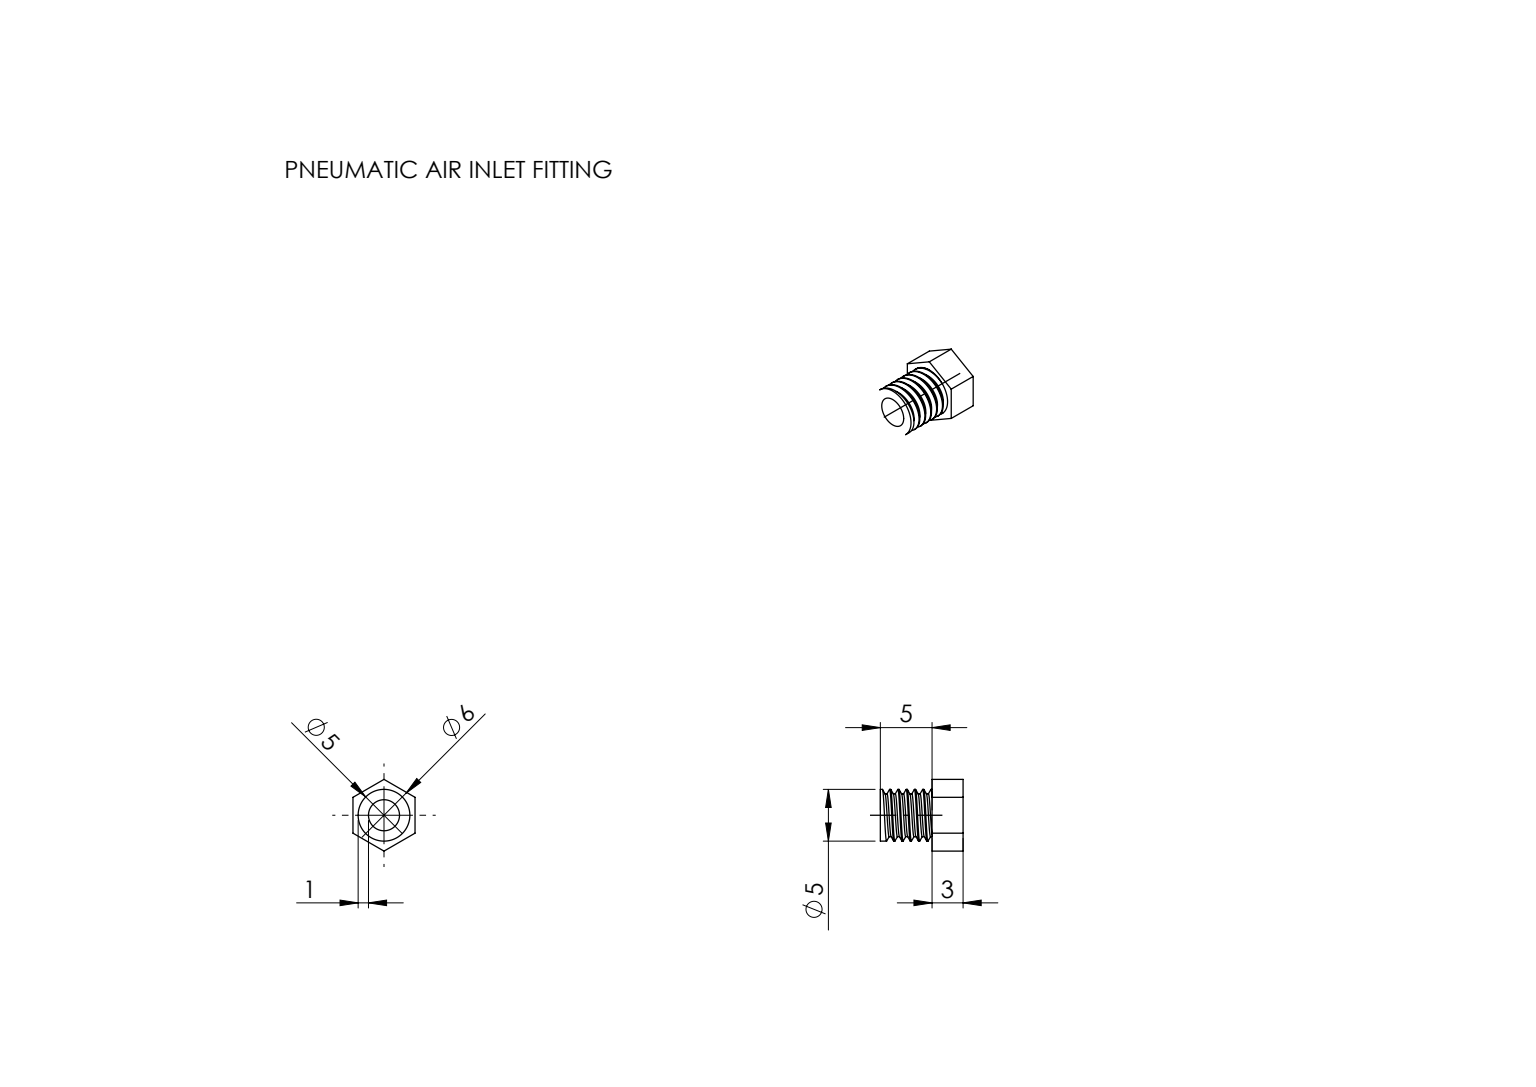
ISO-10303-21;
HEADER;
FILE_DESCRIPTION (('STEP AP214'),
    '1' );
FILE_NAME ('pneumatic air inlet fitting.step',
    '2026-10-04T10:31:01',
    ( '' ),
    ( '' ),
    'SwSTEP 2.0',
    'SolidWorks 2026',
    '' );
FILE_SCHEMA (( 'AUTOMOTIVE_DESIGN' ));
ENDSEC;

DATA;
#1=DIRECTION ( 'NONE',  ( 1.251928832280965695E-16, 1.000000000000000000, 0.000000000000000000 ) ) ;
#9=ORIENTED_EDGE ( 'NONE', *, *, #12350, .T. ) ;
#13=CARTESIAN_POINT ( 'NONE',  ( -1.461580736456472795, 1.461580736456472795, 1.150000001092474688 ) ) ;
#17=CARTESIAN_POINT ( 'NONE',  ( 2.500000000000000000, 3.061616997868383141E-16, 2.100000000000000089 ) ) ;
#21=CARTESIAN_POINT ( 'NONE',  ( 0.8561741729129451750, 2.066987299999999639, 2.000000001092475443 ) ) ;
#26=VERTEX_POINT ( 'NONE', #13779 ) ;
#44=EDGE_LOOP ( 'NONE', ( #13948, #7274 ) ) ;
#48=LINE ( 'NONE', #2436, #232 ) ;
#49=DIRECTION ( 'NONE',  ( -1.000000000000000000, 0.000000000000000000, 0.000000000000000000 ) ) ;
#52=CARTESIAN_POINT ( 'NONE',  ( 1.461580736456473018, -1.461580736456472573, -0.6499999989075253559 ) ) ;
#58=CARTESIAN_POINT ( 'NONE',  ( 0.8561741729129452860, 2.066987299999999639, 2.000000001092474999 ) ) ;
#59=VECTOR ( 'NONE', #8000, 1000.000000000000000 ) ;
#75=CARTESIAN_POINT ( 'NONE',  ( -2.500000000000000000, 0.000000000000000000, -2.199999997815050623 ) ) ;
#81=CARTESIAN_POINT ( 'NONE',  ( 0.000000000000000000, 0.000000000000000000, -5.500000000000000000 ) ) ;
#84=ORIENTED_EDGE ( 'NONE', *, *, #4688, .F. ) ;
#87=ORIENTED_EDGE ( 'NONE', *, *, #14600, .T. ) ;
#88=CARTESIAN_POINT ( 'NONE',  ( -1.035533905932737753, 2.500000000000000444, -1.549999997815050490 ) ) ;
#93=AXIS2_PLACEMENT_3D ( 'NONE', #6041, #2604, #1097 ) ;
#94=CARTESIAN_POINT ( 'NONE',  ( -1.530808498934191571E-16, 2.500000000000000000, 0.6999999999999998446 ) ) ;
#98=CARTESIAN_POINT ( 'NONE',  ( 2.066987299999999639, 0.8561741729129456191, -2.299999998907525711 ) ) ;
#101=DIRECTION ( 'NONE',  ( 0.000000000000000000, 0.000000000000000000, -1.000000000000000000 ) ) ;
#129=CARTESIAN_POINT ( 'NONE',  ( 3.796994071234844259E-16, -2.066987299999999639, 0.8500000010924748661 ) ) ;
#134=CARTESIAN_POINT ( 'NONE',  ( -2.500000000000000000, 0.000000000000000000, -2.199999997815050623 ) ) ;
#136=CARTESIAN_POINT ( 'NONE',  ( 0.8561741729129452860, 2.066987299999999639, -1.199999998907525178 ) ) ;
#139=CARTESIAN_POINT ( 'NONE',  ( 0.8561741729129465073, -2.066987299999999195, 0.7000000010924749549 ) ) ;
#167=CARTESIAN_POINT ( 'NONE',  ( -1.461580736456472351, -1.461580736456473018, -0.2499999989075251672 ) ) ;
#171=CARTESIAN_POINT ( 'NONE',  ( 1.767766952966369320, -1.767766952966368654, 2.000000000000000000 ) ) ;
#175=CARTESIAN_POINT ( 'NONE',  ( 2.066987300000000083, -0.8561741729129449530, -0.7999999989075252671 ) ) ;
#180=ORIENTED_EDGE ( 'NONE', *, *, #12545, .T. ) ;
#187=DIRECTION ( 'NONE',  ( 0.8660254037844385966, 0.4999999999999998890, 0.000000000000000000 ) ) ;
#201=EDGE_CURVE ( 'NONE', #13777, #13408, #2146, .T. ) ;
#202=VERTEX_POINT ( 'NONE', #2611 ) ;
#209=( BOUNDED_CURVE ( )  B_SPLINE_CURVE ( 2, ( #7437, #5274, #15205, #1752, #11093, #14680, #10274, #6626, #3769 ),
 .UNSPECIFIED., .F., .F. ) 
 B_SPLINE_CURVE_WITH_KNOTS ( ( 3, 2, 2, 2, 3 ),
 ( 0.000000000000000000, 0.01785714285714285615, 0.03571428571428571230, 0.05357142857142856845, 0.07142857142857142461 ),
 .UNSPECIFIED. ) 
 CURVE ( )  GEOMETRIC_REPRESENTATION_ITEM ( )  RATIONAL_B_SPLINE_CURVE ( ( 1.000000000000000000, 0.9238795325112867385, 1.000000000000000000, 0.9238795325112867385, 1.000000000000000000, 0.9238795325112867385, 1.000000000000000000, 0.9238795325112867385, 1.000000000000000000 ) ) 
 REPRESENTATION_ITEM ( '' )  );
#213=CARTESIAN_POINT ( 'NONE',  ( 0.8561741729129451750, 2.066987299999999639, -1.199999998907525622 ) ) ;
#220=CARTESIAN_POINT ( 'NONE',  ( -0.8561741729129455081, 2.066987299999999639, -1.899999998907525134 ) ) ;
#222=CARTESIAN_POINT ( 'NONE',  ( -1.265664690411614835E-16, 2.066987299999999639, 0.2500000010924746663 ) ) ;
#232=VECTOR ( 'NONE', #9608, 1000.000000000000000 ) ;
#248=CARTESIAN_POINT ( 'NONE',  ( 3.796994071234844259E-16, -2.066987299999999639, -0.1499999989075253282 ) ) ;
#252=CARTESIAN_POINT ( 'NONE',  ( 0.4831378333609244180, 2.500000000000000000, -2.516327958217759342 ) ) ;
#256=CARTESIAN_POINT ( 'NONE',  ( 3.796994071234844259E-16, -2.066987299999999639, 0.8500000010924748661 ) ) ;
#286=CARTESIAN_POINT ( 'NONE',  ( -0.8561741729129455081, 2.066987299999999639, -1.899999998907525134 ) ) ;
#289=ADVANCED_FACE ( 'NONE', ( #4509 ), #10713, .T. ) ;
#294=LINE ( 'NONE', #13810, #11835 ) ;
#325=CARTESIAN_POINT ( 'NONE',  ( -2.066987299999999639, 0.8561741729129452860, 0.4000000010924749105 ) ) ;
#326=CARTESIAN_POINT ( 'NONE',  ( -1.767766952966369098, 1.767766952966369098, -1.600000000000000311 ) ) ;
#329=CARTESIAN_POINT ( 'NONE',  ( -2.500000000000000444, 1.035533905932737753, 0.05000000000000014155 ) ) ;
#333=CARTESIAN_POINT ( 'NONE',  ( 0.8561741729129451750, 2.066987299999999639, -1.199999998907525622 ) ) ;
#338=VERTEX_POINT ( 'NONE', #15412 ) ;
#355=EDGE_CURVE ( 'NONE', #9607, #3437, #6727, .T. ) ;
#360=CARTESIAN_POINT ( 'NONE',  ( -2.500000000000000000, 0.000000000000000000, 1.700000000000000178 ) ) ;
#366=CARTESIAN_POINT ( 'NONE',  ( -1.265664690411614835E-16, 2.066987299999999639, -1.149999998907525356 ) ) ;
#372=CARTESIAN_POINT ( 'NONE',  ( 2.066987300000000083, -0.8561741729129450640, -1.399999998907525134 ) ) ;
#373=CARTESIAN_POINT ( 'NONE',  ( 2.500000000000000000, 3.061616997868383141E-16, -2.599999997815050534 ) ) ;
#374=CARTESIAN_POINT ( 'NONE',  ( 0.8561741729129452860, 2.066987299999999639, 1.800000001092475044 ) ) ;
#379=CARTESIAN_POINT ( 'NONE',  ( 2.500000000000000000, 3.061616997868383141E-16, -0.2999999999999999334 ) ) ;
#399=CARTESIAN_POINT ( 'NONE',  ( 2.066987299999999639, 0.8561741729129456191, -2.299999998907525711 ) ) ;
#403=CARTESIAN_POINT ( 'NONE',  ( -2.500000000000000000, 0.000000000000000000, 1.800000002184949821 ) ) ;
#406=CARTESIAN_POINT ( 'NONE',  ( 1.035533905932737531, 2.500000000000000444, -0.8499999978150500901 ) ) ;
#407=CARTESIAN_POINT ( 'NONE',  ( 3.796994071234844259E-16, -2.066987299999999639, 0.05000000109247476621 ) ) ;
#408=( BOUNDED_CURVE ( )  B_SPLINE_CURVE ( 2, ( #13845, #5357, #15207, #15052, #7888, #406, #8045, #8938, #10125 ),
 .UNSPECIFIED., .F., .F. ) 
 B_SPLINE_CURVE_WITH_KNOTS ( ( 3, 2, 2, 2, 3 ),
 ( 0.4285714285714285476, 0.4464285714285714524, 0.4642857142857143016, 0.4821428571428571508, 0.5000000000000000000 ),
 .UNSPECIFIED. ) 
 CURVE ( )  GEOMETRIC_REPRESENTATION_ITEM ( )  RATIONAL_B_SPLINE_CURVE ( ( 1.000000000000000000, 0.9238795325112867385, 1.000000000000000000, 0.9238795325112867385, 1.000000000000000000, 0.9238795325112867385, 1.000000000000000000, 0.9238795325112867385, 1.000000000000000000 ) ) 
 REPRESENTATION_ITEM ( '' )  );
#412=EDGE_LOOP ( 'NONE', ( #8229, #15228, #15119, #15116 ) ) ;
#413=VECTOR ( 'NONE', #15523, 1000.000000000000000 ) ;
#439=CARTESIAN_POINT ( 'NONE',  ( 1.035533905932737531, 2.500000000000000444, 1.450000000000000400 ) ) ;
#477=APPLICATION_CONTEXT ( 'automotive_design' ) ;
#480=CARTESIAN_POINT ( 'NONE',  ( 2.066987300000000083, -0.8561741729129449530, -2.399999998907525356 ) ) ;
#483=CARTESIAN_POINT ( 'NONE',  ( 1.767766952966369320, -1.767766952966368654, -0.4000000000000001887 ) ) ;
#487=CARTESIAN_POINT ( 'NONE',  ( -1.265664690411614835E-16, 2.066987299999999639, -1.149999998907525356 ) ) ;
#503=CARTESIAN_POINT ( 'NONE',  ( 1.767766952966369320, -1.767766952966368654, -2.000000000000000444 ) ) ;
#510=CARTESIAN_POINT ( 'NONE',  ( -2.055837405312323174, -1.429616716009805888, -2.499172079278979997 ) ) ;
#519=CARTESIAN_POINT ( 'NONE',  ( 1.461580736456472573, 1.461580736456472795, -1.249999998907525223 ) ) ;
#528=CARTESIAN_POINT ( 'NONE',  ( -0.8561741729129458411, -2.066987299999999195, -1.799999998907525045 ) ) ;
#546=VERTEX_POINT ( 'NONE', #7374 ) ;
#553=EDGE_CURVE ( 'NONE', #3385, #10225, #2858, .T. ) ;
#556=CARTESIAN_POINT ( 'NONE',  ( -3.000000000000000444, -1.732050807568878081, -5.500000000000000000 ) ) ;
#560=CARTESIAN_POINT ( 'NONE',  ( -1.035533905932737753, 2.500000000000000444, -0.05000000000000014155 ) ) ;
#564=DIRECTION ( 'NONE',  ( 0.000000000000000000, 0.000000000000000000, 1.000000000000000000 ) ) ;
#565=CARTESIAN_POINT ( 'NONE',  ( -1.461580736456472795, 1.461580736456472795, -0.2499999989075251672 ) ) ;
#573=ORIENTED_EDGE ( 'NONE', *, *, #355, .F. ) ;
#575=CARTESIAN_POINT ( 'NONE',  ( 1.035533905932739085, -2.500000000000000000, 0.4500000021849495657 ) ) ;
#587=EDGE_LOOP ( 'NONE', ( #4059, #13067, #6384, #6203 ) ) ;
#598=CARTESIAN_POINT ( 'NONE',  ( -2.500000000000000000, -1.035533905932739307, -0.6500000000000000222 ) ) ;
#605=CARTESIAN_POINT ( 'NONE',  ( 2.066987299999999639, 2.531329380823229670E-16, -1.549999998907525489 ) ) ;
#631=DIRECTION ( 'NONE',  ( -0.8660254037844387076, -0.4999999999999998890, 0.000000000000000000 ) ) ;
#632=CARTESIAN_POINT ( 'NONE',  ( 1.035533905932737531, 2.500000000000000444, -1.750000000000000222 ) ) ;
#646=CARTESIAN_POINT ( 'NONE',  ( 4.592425496802573972E-16, -2.500000000000000000, 0.4000000021849496878 ) ) ;
#654=CARTESIAN_POINT ( 'NONE',  ( -1.265664690411614835E-16, 2.066987299999999639, 1.850000001092474644 ) ) ;
#659=CARTESIAN_POINT ( 'NONE',  ( 2.356441885422377425, -0.8834023615831587684, -2.499692266475796121 ) ) ;
#669=CARTESIAN_POINT ( 'NONE',  ( 1.035533905932739085, -2.500000000000000000, -0.4499999999999998446 ) ) ;
#679=CARTESIAN_POINT ( 'NONE',  ( -2.066987299999999195, -0.8561741729129467293, -1.099999998907525312 ) ) ;
#685=ORIENTED_EDGE ( 'NONE', *, *, #2400, .T. ) ;
#707=CARTESIAN_POINT ( 'NONE',  ( -0.8561741729129458411, -2.066987299999999195, -2.599999998907525534 ) ) ;
#713=CARTESIAN_POINT ( 'NONE',  ( 4.592425496802573972E-16, -2.500000000000000000, -0.5000000000000000000 ) ) ;
#715=CARTESIAN_POINT ( 'NONE',  ( 2.500000000000000000, 3.061616997868383141E-16, -1.799999997815050490 ) ) ;
#720=ADVANCED_FACE ( 'NONE', ( #5682 ), #7733, .T. ) ;
#726=PLANE ( 'NONE',  #3772 ) ;
#730=CARTESIAN_POINT ( 'NONE',  ( -2.500000000000000444, 1.035533905932737753, 0.1500000021849496601 ) ) ;
#735=CARTESIAN_POINT ( 'NONE',  ( -2.500000000000000000, 0.000000000000000000, 1.706999999978150662 ) ) ;
#737=SHAPE_DEFINITION_REPRESENTATION ( #15269, #5305 ) ;
#739=CARTESIAN_POINT ( 'NONE',  ( -1.265664690411614835E-16, 2.066987299999999639, 0.2500000010924746663 ) ) ;
#743=CARTESIAN_POINT ( 'NONE',  ( -1.530808498934191571E-16, 2.500000000000000000, 0.8000000021849498211 ) ) ;
#745=CARTESIAN_POINT ( 'NONE',  ( -2.135032056815611146, -1.308652412870009663, -2.499304978889202555 ) ) ;
#753=CARTESIAN_POINT ( 'NONE',  ( 0.3272492347489360798, 2.500000000000000000, -2.500000000000000000 ) ) ;
#755=CARTESIAN_POINT ( 'NONE',  ( 2.500000000000000444, 1.035533905932737975, -1.850000000000000533 ) ) ;
#765=CARTESIAN_POINT ( 'NONE',  ( 1.461580736456473018, -1.461580736456472573, -0.04999999890752549608 ) ) ;
#771=EDGE_CURVE ( 'NONE', #5999, #10225, #9169, .T. ) ;
#776=CARTESIAN_POINT ( 'NONE',  ( 4.592425496802573972E-16, -2.500000000000000000, -0.3999999978150502455 ) ) ;
#782=CARTESIAN_POINT ( 'NONE',  ( -1.035533905932738197, -2.500000000000000000, 1.150000002184949466 ) ) ;
#786=VERTEX_POINT ( 'NONE', #4622 ) ;
#794=CARTESIAN_POINT ( 'NONE',  ( -2.500000000000000000, -1.035533905932739307, -0.5499999978150503788 ) ) ;
#801=ORIENTED_EDGE ( 'NONE', *, *, #1804, .T. ) ;
#805=PLANE ( 'NONE',  #9364 ) ;
#808=CARTESIAN_POINT ( 'NONE',  ( 2.500000000000000000, 3.061616997868383141E-16, 0.6000000021849495324 ) ) ;
#812=CARTESIAN_POINT ( 'NONE',  ( -1.530808498934191571E-16, 2.500000000000000000, -1.693000000021849916 ) ) ;
#815=CARTESIAN_POINT ( 'NONE',  ( -1.265664690411614835E-16, 2.066987299999999639, 1.050000001092474822 ) ) ;
#822=CARTESIAN_POINT ( 'NONE',  ( -2.397391504966196241, 0.7648662538461182825, -2.499399845735361225 ) ) ;
#833=CARTESIAN_POINT ( 'NONE',  ( 2.500000000000000444, 1.035533905932737975, 0.5499999999999999334 ) ) ;
#836=( BOUNDED_CURVE ( )  B_SPLINE_CURVE ( 2, ( #3676, #14327, #3434, #8554, #13378 ),
 .UNSPECIFIED., .F., .F. ) 
 B_SPLINE_CURVE_WITH_KNOTS ( ( 3, 2, 3 ),
 ( 0.8571428571428570953, 0.8750000000000000000, 0.8928571428571429047 ),
 .UNSPECIFIED. ) 
 CURVE ( )  GEOMETRIC_REPRESENTATION_ITEM ( )  RATIONAL_B_SPLINE_CURVE ( ( 1.000000000000000000, 0.9238795325112867385, 1.000000000000000000, 0.9238795325112867385, 1.000000000000000000 ) ) 
 REPRESENTATION_ITEM ( '' )  );
#848=CARTESIAN_POINT ( 'NONE',  ( 0.000000000000000000, 0.000000000000000000, 2.500000000000000000 ) ) ;
#870=CARTESIAN_POINT ( 'NONE',  ( -1.035533905932738197, -2.500000000000000000, 1.150000002184949466 ) ) ;
#873=CARTESIAN_POINT ( 'NONE',  ( -2.500000000000000000, 0.000000000000000000, 0.9000000000000000222 ) ) ;
#879=ORIENTED_EDGE ( 'NONE', *, *, #5328, .F. ) ;
#883=CARTESIAN_POINT ( 'NONE',  ( -2.500000000000000000, -1.035533905932739307, -0.5499999978150504898 ) ) ;
#887=CARTESIAN_POINT ( 'NONE',  ( 1.035533905932739085, -2.500000000000000000, -0.4430000000218494716 ) ) ;
#890=CARTESIAN_POINT ( 'NONE',  ( 1.461580736456473018, -1.461580736456472573, 1.550000001092474822 ) ) ;
#900=LINE ( 'NONE', #8075, #8869 ) ;
#908=CARTESIAN_POINT ( 'NONE',  ( -2.500000000000000000, -1.035533905932739307, 0.9499999999999999556 ) ) ;
#914=( BOUNDED_CURVE ( )  B_SPLINE_CURVE ( 2, ( #2367, #1402, #6046, #2449, #8594, #10887, #8350, #11039, #13269 ),
 .UNSPECIFIED., .F., .F. ) 
 B_SPLINE_CURVE_WITH_KNOTS ( ( 3, 2, 2, 2, 3 ),
 ( 0.1428571428571428492, 0.1607142857142857262, 0.1785714285714285754, 0.1964285714285714246, 0.2142857142857142738 ),
 .UNSPECIFIED. ) 
 CURVE ( )  GEOMETRIC_REPRESENTATION_ITEM ( )  RATIONAL_B_SPLINE_CURVE ( ( 1.000000000000000000, 0.9238795325112867385, 1.000000000000000000, 0.9238795325112867385, 1.000000000000000000, 0.9238795325112867385, 1.000000000000000000, 0.9238795325112867385, 1.000000000000000000 ) ) 
 REPRESENTATION_ITEM ( '' )  );
#922=ORIENTED_EDGE ( 'NONE', *, *, #11635, .F. ) ;
#930=AXIS2_PLACEMENT_3D ( 'NONE', #4602, #8185, #8263 ) ;
#933=CARTESIAN_POINT ( 'NONE',  ( 1.461580736456473018, -1.461580736456472573, 1.750000001092474999 ) ) ;
#941=ORIENTED_EDGE ( 'NONE', *, *, #5328, .T. ) ;
#948=FACE_OUTER_BOUND ( 'NONE', #587, .T. ) ;
#949=CARTESIAN_POINT ( 'NONE',  ( -2.500000000000000444, 1.035533905932737753, -0.6499999978150502455 ) ) ;
#953=CARTESIAN_POINT ( 'NONE',  ( -1.767766952966369098, 1.767766952966369098, 0.7999999999999999334 ) ) ;
#964=CARTESIAN_POINT ( 'NONE',  ( 2.066987300000000083, -0.8561741729129449530, 1.600000001092474644 ) ) ;
#969=CARTESIAN_POINT ( 'NONE',  ( -1.530808498934191571E-16, 2.500000000000000000, -0.8930000000218497602 ) ) ;
#972=CARTESIAN_POINT ( 'NONE',  ( 0.8561741729129463963, -2.066987299999999195, 1.500000001092474555 ) ) ;
#987=CYLINDRICAL_SURFACE ( 'NONE', #1712, 2.500000000000000000 ) ;
#1003=CARTESIAN_POINT ( 'NONE',  ( -1.767766952966369098, 1.767766952966369098, -1.499999997815050001 ) ) ;
#1009=CARTESIAN_POINT ( 'NONE',  ( -2.066987299999999639, 0.8561741729129452860, 1.400000001092474911 ) ) ;
#1017=CARTESIAN_POINT ( 'NONE',  ( -1.461580736456472795, 1.461580736456472795, -1.049999998907525045 ) ) ;
#1018=CARTESIAN_POINT ( 'NONE',  ( -2.500000000000000000, 0.000000000000000000, -1.399999997815050357 ) ) ;
#1029=CARTESIAN_POINT ( 'NONE',  ( 1.035533905932737531, 2.500000000000000444, -1.649999997815050357 ) ) ;
#1045=CARTESIAN_POINT ( 'NONE',  ( -2.500000000000000444, 1.035533905932737753, -1.449999997815050623 ) ) ;
#1049=CARTESIAN_POINT ( 'NONE',  ( 1.035533905932737531, 2.500000000000000444, -0.9430000000218496936 ) ) ;
#1052=CARTESIAN_POINT ( 'NONE',  ( -1.265664690411614835E-16, 2.066987299999999639, -2.149999998907525800 ) ) ;
#1057=VECTOR ( 'NONE', #10344, 1000.000000000000000 ) ;
#1084=CARTESIAN_POINT ( 'NONE',  ( 2.500000000000000000, 3.061616997868383141E-16, -1.100000000000000311 ) ) ;
#1089=CARTESIAN_POINT ( 'NONE',  ( 1.461580736456472573, 1.461580736456472795, 1.150000001092474911 ) ) ;
#1096=CARTESIAN_POINT ( 'NONE',  ( -2.066987299999999195, -0.8561741729129467293, 1.500000001092474777 ) ) ;
#1097=DIRECTION ( 'NONE',  ( -1.000000000000000000, 0.000000000000000000, 0.000000000000000000 ) ) ;
#1110=CARTESIAN_POINT ( 'NONE',  ( -2.500000000000000444, 1.035533905932737753, 0.9500000021849498433 ) ) ;
#1122=CARTESIAN_POINT ( 'NONE',  ( -1.265664690411614835E-16, 2.066987299999999639, 1.050000001092474822 ) ) ;
#1126=CARTESIAN_POINT ( 'NONE',  ( -1.767766952966369098, 1.767766952966369098, 0.006999999978150502240 ) ) ;
#1129=CARTESIAN_POINT ( 'NONE',  ( -1.461580736456472351, -1.461580736456473018, -2.649999998907525356 ) ) ;
#1134=ORIENTED_EDGE ( 'NONE', *, *, #3829, .F. ) ;
#1143=EDGE_CURVE ( 'NONE', #8784, #13466, #6997, .T. ) ;
#1163=CARTESIAN_POINT ( 'NONE',  ( 2.066987300000000083, -0.8561741729129449530, 0.2000000010924747329 ) ) ;
#1171=CARTESIAN_POINT ( 'NONE',  ( -2.066987299999999639, 0.000000000000000000, -0.1499999989075253282 ) ) ;
#1191=ORIENTED_EDGE ( 'NONE', *, *, #15384, .T. ) ;
#1197=CARTESIAN_POINT ( 'NONE',  ( -1.767766952966369098, 1.767766952966369098, -3.099999997815050090 ) ) ;
#1202=CARTESIAN_POINT ( 'NONE',  ( 1.035533905932739085, -2.500000000000000000, 1.949999999999999956 ) ) ;
#1206=CARTESIAN_POINT ( 'NONE',  ( 1.461580736456472573, 1.461580736456472795, -1.449999998907525178 ) ) ;
#1214=VERTEX_POINT ( 'NONE', #12948 ) ;
#1219=DIRECTION ( 'NONE',  ( 0.5000000000000001110, 0.8660254037844385966, 0.000000000000000000 ) ) ;
#1223=CARTESIAN_POINT ( 'NONE',  ( 0.000000000000000000, 0.000000000000000000, 2.500000000000000000 ) ) ;
#1242=EDGE_CURVE ( 'NONE', #5900, #7812, #3452, .T. ) ;
#1244=CARTESIAN_POINT ( 'NONE',  ( -0.8561741729129458411, -2.066987299999999195, -0.7999999989075252671 ) ) ;
#1250=CARTESIAN_POINT ( 'NONE',  ( 1.461580736456472573, 1.461580736456472795, 0.3500000010924749216 ) ) ;
#1259=VECTOR ( 'NONE', #15235, 1000.000000000000227 ) ;
#1264=CARTESIAN_POINT ( 'NONE',  ( -2.500000000000000444, 1.035533905932737753, -3.049999997815050268 ) ) ;
#1270=ORIENTED_EDGE ( 'NONE', *, *, #12295, .F. ) ;
#1273=ORIENTED_EDGE ( 'NONE', *, *, #3458, .F. ) ;
#1274=EDGE_CURVE ( 'NONE', #2475, #11794, #294, .T. ) ;
#1278=CARTESIAN_POINT ( 'NONE',  ( 2.500000000000000000, 3.061616997868383141E-16, -2.599999997815050534 ) ) ;
#1282=CARTESIAN_POINT ( 'NONE',  ( 2.500000000000000444, 1.035533905932737975, 2.149999999999999911 ) ) ;
#1286=CARTESIAN_POINT ( 'NONE',  ( 1.461580736456473018, -1.461580736456472573, -2.449999998907525622 ) ) ;
#1290=VERTEX_POINT ( 'NONE', #6516 ) ;
#1318=CARTESIAN_POINT ( 'NONE',  ( 2.066987299999999639, 2.531329380823229670E-16, 1.850000001092474866 ) ) ;
#1320=ADVANCED_FACE ( 'NONE', ( #2764, #8667 ), #14937, .F. ) ;
#1321=LINE ( 'NONE', #6197, #2164 ) ;
#1326=CARTESIAN_POINT ( 'NONE',  ( -0.8561741729129455081, 2.066987299999999639, -2.699999998907525622 ) ) ;
#1343=CARTESIAN_POINT ( 'NONE',  ( -2.500000000000000000, 0.000000000000000000, -2.999999997815050889 ) ) ;
#1344=DIRECTION ( 'NONE',  ( 0.000000000000000000, 0.000000000000000000, 1.000000000000000000 ) ) ;
#1351=EDGE_LOOP ( 'NONE', ( #3419, #1134, #3681, #13778, #10714 ) ) ;
#1356=CARTESIAN_POINT ( 'NONE',  ( -1.461580736456472795, 1.461580736456472795, 0.3500000010924746996 ) ) ;
#1361=CARTESIAN_POINT ( 'NONE',  ( -1.035533905932737753, 2.500000000000000444, 1.550000000000000044 ) ) ;
#1365=CARTESIAN_POINT ( 'NONE',  ( -0.8561741729129458411, -2.066987299999999195, -0.9999999989075254447 ) ) ;
#1387=ORIENTED_EDGE ( 'NONE', *, *, #10097, .T. ) ;
#1390=CARTESIAN_POINT ( 'NONE',  ( -1.530808498934191571E-16, 2.500000000000000000, -0.9000000000000002442 ) ) ;
#1394=CARTESIAN_POINT ( 'NONE',  ( -1.461580736456472351, -1.461580736456473018, -2.449999998907525178 ) ) ;
#1402=CARTESIAN_POINT ( 'NONE',  ( -2.500000000000000444, 1.035533905932737753, 1.649999999999999911 ) ) ;
#1417=LINE ( 'NONE', #14557, #14169 ) ;
#1425=( BOUNDED_CURVE ( )  B_SPLINE_CURVE ( 2, ( #5701, #11576, #12925, #9201, #13963, #3070, #14041, #7921, #15403 ),
 .UNSPECIFIED., .F., .F. ) 
 B_SPLINE_CURVE_WITH_KNOTS ( ( 3, 2, 2, 2, 3 ),
 ( 0.000000000000000000, 0.01785714285714285615, 0.03571428571428571230, 0.05357142857142856845, 0.07142857142857142461 ),
 .UNSPECIFIED. ) 
 CURVE ( )  GEOMETRIC_REPRESENTATION_ITEM ( )  RATIONAL_B_SPLINE_CURVE ( ( 1.000000000000000000, 0.9238795325112867385, 1.000000000000000000, 0.9238795325112867385, 1.000000000000000000, 0.9238795325112867385, 1.000000000000000000, 0.9238795325112867385, 1.000000000000000000 ) ) 
 REPRESENTATION_ITEM ( '' )  );
#1431=CARTESIAN_POINT ( 'NONE',  ( 0.8561741729129451750, 2.066987299999999639, -1.399999998907525800 ) ) ;
#1436=CARTESIAN_POINT ( 'NONE',  ( -2.500000000000000444, 1.035533905932737753, 2.449999999999999734 ) ) ;
#1439=CARTESIAN_POINT ( 'NONE',  ( -2.066987299999999639, 0.8561741729129452860, 0.6000000010924748661 ) ) ;
#1475=CARTESIAN_POINT ( 'NONE',  ( -2.066987299999999639, 0.8561741729129452860, -1.799999998907525267 ) ) ;
#1479=CARTESIAN_POINT ( 'NONE',  ( -2.283493650000000041, 0.000000000000000000, 2.375000000546237278 ) ) ;
#1481=CARTESIAN_POINT ( 'NONE',  ( 0.8561741729129452860, 2.066987299999999639, -1.999999998907525445 ) ) ;
#1482=CARTESIAN_POINT ( 'NONE',  ( -1.035533905932737753, 2.500000000000000444, -3.149999997815050801 ) ) ;
#1483=CARTESIAN_POINT ( 'NONE',  ( -2.066987299999999639, 0.000000000000000000, 2.050000001092474822 ) ) ;
#1513=CARTESIAN_POINT ( 'NONE',  ( -0.8561741729129458411, -2.066987299999999195, -0.9999999989075254447 ) ) ;
#1517=CARTESIAN_POINT ( 'NONE',  ( -2.500000000000000000, 0.000000000000000000, 0.09999999999999982514 ) ) ;
#1520=MECHANICAL_DESIGN_GEOMETRIC_PRESENTATION_REPRESENTATION('',(#15246),#9915);
#1522=CARTESIAN_POINT ( 'NONE',  ( 2.066987299999999639, 2.531329380823229670E-16, -0.5499999989075250451 ) ) ;
#1556=CARTESIAN_POINT ( 'NONE',  ( 1.035533905932739085, -2.500000000000000000, 1.150000000000000133 ) ) ;
#1563=CARTESIAN_POINT ( 'NONE',  ( 0.000000000000000000, 0.000000000000000000, -2.500000000000000000 ) ) ;
#1565=CARTESIAN_POINT ( 'NONE',  ( -1.767766952966368432, -1.767766952966369320, -2.899999997815050357 ) ) ;
#1566=CARTESIAN_POINT ( 'NONE',  ( 2.066987300000000083, -0.8561741729129450640, 1.092474635061568626E-09 ) ) ;
#1570=VERTEX_POINT ( 'NONE', #10257 ) ;
#1575=CARTESIAN_POINT ( 'NONE',  ( -2.500000000000000000, 0.000000000000000000, 0.09999999999999982514 ) ) ;
#1591=CARTESIAN_POINT ( 'NONE',  ( 0.8561741729129451750, 2.066987299999999639, -2.199999998907525622 ) ) ;
#1595=CARTESIAN_POINT ( 'NONE',  ( 0.9662756667218489470, 2.500000000000000000, -2.546655916391819652 ) ) ;
#1598=CARTESIAN_POINT ( 'NONE',  ( -1.461580736456472795, 1.461580736456472795, 0.5500000010924748217 ) ) ;
#1603=ORIENTED_EDGE ( 'NONE', *, *, #7772, .F. ) ;
#1616=CARTESIAN_POINT ( 'NONE',  ( 2.500000000000000444, 1.035533905932737975, 1.356999999978150573 ) ) ;
#1624=ORIENTED_EDGE ( 'NONE', *, *, #4651, .T. ) ;
#1633=CARTESIAN_POINT ( 'NONE',  ( 1.767766952966369320, -1.767766952966368654, 2.000000000000000000 ) ) ;
#1636=CARTESIAN_POINT ( 'NONE',  ( -1.035533905932738197, -2.500000000000000000, -0.5500000000000001554 ) ) ;
#1639=CARTESIAN_POINT ( 'NONE',  ( 2.066987299999999639, 0.8561741729129456191, -2.099999998907525534 ) ) ;
#1642=CARTESIAN_POINT ( 'NONE',  ( 0.8561741729129452860, 2.066987299999999639, 1.000000001092474555 ) ) ;
#1649=ADVANCED_FACE ( 'NONE', ( #12149 ), #14287, .T. ) ;
#1651=DIRECTION ( 'NONE',  ( 1.000000000000000000, 0.000000000000000000, 0.000000000000000000 ) ) ;
#1668=CARTESIAN_POINT ( 'NONE',  ( -1.265664690411614835E-16, 2.066987299999999639, 0.2500000010924746663 ) ) ;
#1672=CARTESIAN_POINT ( 'NONE',  ( 2.500000000000000000, 3.061616997868383141E-16, -1.100000000000000311 ) ) ;
#1676=CARTESIAN_POINT ( 'NONE',  ( -0.8561741729129455081, 2.066987299999999639, -1.099999998907525089 ) ) ;
#1698=EDGE_LOOP ( 'NONE', ( #15231, #87, #3481, #13122 ) ) ;
#1699=CARTESIAN_POINT ( 'NONE',  ( 2.460891429721819179, -0.4634845133093605241, -2.499202848233824881 ) ) ;
#1707=CARTESIAN_POINT ( 'NONE',  ( 1.767766952966368654, 1.767766952966369098, 1.399999999999999911 ) ) ;
#1709=EDGE_CURVE ( 'NONE', #202, #338, #11413, .T. ) ;
#1712=AXIS2_PLACEMENT_3D ( 'NONE', #13073, #8239, #10852 ) ;
#1713=EDGE_CURVE ( 'NONE', #10824, #5765, #15504, .T. ) ;
#1718=CARTESIAN_POINT ( 'NONE',  ( 3.796994071234844259E-16, -2.066987299999999639, -0.9499999989075252893 ) ) ;
#1747=CARTESIAN_POINT ( 'NONE',  ( 0.8561741729129463963, -2.066987299999999195, -2.499999998907525445 ) ) ;
#1751=CARTESIAN_POINT ( 'NONE',  ( 1.767766952966368654, 1.767766952966369098, 1.500000002184949777 ) ) ;
#1752=CARTESIAN_POINT ( 'NONE',  ( -1.035533905932737753, 2.500000000000000444, 2.350000000000000533 ) ) ;
#1756=CARTESIAN_POINT ( 'NONE',  ( -2.066987299999999639, 0.8561741729129452860, -1.799999998907525267 ) ) ;
#1766=CARTESIAN_POINT ( 'NONE',  ( -1.767766952966369098, 1.767766952966369098, 0.1000000021849495324 ) ) ;
#1768=COLOUR_RGB ( '', 0.31764706, 0.68627451, 0.89019608) ;
#1788=CARTESIAN_POINT ( 'NONE',  ( 2.500000000000000000, 3.061616997868383141E-16, 0.5000000000000000000 ) ) ;
#1796=CARTESIAN_POINT ( 'NONE',  ( 2.066987300000000083, -0.8561741729129450640, -1.599999998907525756 ) ) ;
#1804=EDGE_CURVE ( 'NONE', #5264, #3385, #3580, .T. ) ;
#1813=CARTESIAN_POINT ( 'NONE',  ( -2.066987299999999639, 0.8561741729129455081, 2.200000001092474733 ) ) ;
#1822=CARTESIAN_POINT ( 'NONE',  ( -1.530808498934191571E-16, 2.500000000000000000, -3.199999997815050623 ) ) ;
#1825=CARTESIAN_POINT ( 'NONE',  ( 3.796994071234844259E-16, -2.066987299999999639, -2.549999998907525267 ) ) ;
#1828=CARTESIAN_POINT ( 'NONE',  ( -1.767766952966369098, 1.767766952966369098, 0.000000000000000000 ) ) ;
#1832=CARTESIAN_POINT ( 'NONE',  ( 2.066987299999999639, 2.531329380823229670E-16, -2.149999998907525356 ) ) ;
#1842=CARTESIAN_POINT ( 'NONE',  ( 1.767766952966369320, -1.767766952966368654, 0.5000000021849494436 ) ) ;
#1846=ADVANCED_FACE ( 'NONE', ( #14780 ), #13571, .F. ) ;
#1848=CARTESIAN_POINT ( 'NONE',  ( -2.500000000000000000, -0.9567085809127248153, 2.553193976603714610 ) ) ;
#1850=PRODUCT_CONTEXT ( 'NONE', #477, 'mechanical' ) ;
#1853=EDGE_CURVE ( 'NONE', #3437, #2475, #6220, .T. ) ;
#1857=CARTESIAN_POINT ( 'NONE',  ( -1.798270642782740181, 1.742470094454686036, -2.500251818840280471 ) ) ;
#1858=VECTOR ( 'NONE', #12170, 1000.000000000000000 ) ;
#1861=DIRECTION ( 'NONE',  ( 0.000000000000000000, 0.000000000000000000, 1.000000000000000000 ) ) ;
#1865=CARTESIAN_POINT ( 'NONE',  ( 1.035533905932739085, -2.500000000000000000, 1.949999999999999956 ) ) ;
#1866=CARTESIAN_POINT ( 'NONE',  ( -1.767766952966368432, -1.767766952966369320, -1.400000000000000133 ) ) ;
#1874=CARTESIAN_POINT ( 'NONE',  ( 0.8561741729129452860, 2.066987299999999639, -2.199999998907525622 ) ) ;
#1897=VERTEX_POINT ( 'NONE', #5154 ) ;
#1904=CARTESIAN_POINT ( 'NONE',  ( -1.767766952966368432, -1.767766952966369320, -0.6000000000000003109 ) ) ;
#1905=CARTESIAN_POINT ( 'NONE',  ( 2.500000000000000444, -1.035533905932737309, -1.149999999999999689 ) ) ;
#1906=VECTOR ( 'NONE', #7020, 1000.000000000000000 ) ;
#1915=EDGE_LOOP ( 'NONE', ( #1624, #4932, #12716, #2964 ) ) ;
#1917=FACE_OUTER_BOUND ( 'NONE', #13307, .T. ) ;
#1921=CARTESIAN_POINT ( 'NONE',  ( 1.767766952966369320, -1.767766952966368654, -0.2999999978150506563 ) ) ;
#1925=CARTESIAN_POINT ( 'NONE',  ( -1.035533905932738197, -2.500000000000000000, 1.856999999978150573 ) ) ;
#1928=CARTESIAN_POINT ( 'NONE',  ( -0.8561741729129455081, 2.066987299999999639, 0.3000000010924747662 ) ) ;
#1933=CARTESIAN_POINT ( 'NONE',  ( 2.383412885783723123, 0.8083228232074107789, -2.500305643928210309 ) ) ;
#1941=CARTESIAN_POINT ( 'NONE',  ( -2.500000000000000000, 0.000000000000000000, 2.500000000000000000 ) ) ;
#1942=CARTESIAN_POINT ( 'NONE',  ( 0.6543697108982007293, 2.434931691670788823, -2.500000000000000000 ) ) ;
#1943=CARTESIAN_POINT ( 'NONE',  ( -1.530808498934191571E-16, 2.500000000000000000, -1.700000000000000622 ) ) ;
#1945=( LENGTH_UNIT ( ) NAMED_UNIT ( * ) SI_UNIT ( .MILLI., .METRE. ) );
#1948=( BOUNDED_CURVE ( )  B_SPLINE_CURVE ( 2, ( #4139, #9162, #326, #13686, #7882, #10196, #3976, #2716, #13841 ),
 .UNSPECIFIED., .F., .F. ) 
 B_SPLINE_CURVE_WITH_KNOTS ( ( 3, 2, 2, 2, 3 ),
 ( 0.7142857142857143016, 0.7321428571428570953, 0.7500000000000000000, 0.7678571428571429047, 0.7857142857142856984 ),
 .UNSPECIFIED. ) 
 CURVE ( )  GEOMETRIC_REPRESENTATION_ITEM ( )  RATIONAL_B_SPLINE_CURVE ( ( 1.000000000000000000, 0.9238795325112867385, 1.000000000000000000, 0.9238795325112867385, 1.000000000000000000, 0.9238795325112867385, 1.000000000000000000, 0.9238795325112867385, 1.000000000000000000 ) ) 
 REPRESENTATION_ITEM ( '' )  );
#1953=CARTESIAN_POINT ( 'NONE',  ( -2.066987299999999195, -0.8561741729129467293, -2.699999998907525178 ) ) ;
#1969=CARTESIAN_POINT ( 'NONE',  ( 1.035533905932739085, -2.500000000000000000, 1.250000002184949999 ) ) ;
#1970=ORIENTED_EDGE ( 'NONE', *, *, #9346, .T. ) ;
#1976=EDGE_CURVE ( 'NONE', #15372, #15063, #4775, .T. ) ;
#1985=CARTESIAN_POINT ( 'NONE',  ( 1.035533905932737531, 2.500000000000000444, -0.04999999781505021224 ) ) ;
#1998=CARTESIAN_POINT ( 'NONE',  ( 1.767766952966368654, 1.767766952966369098, -0.09999999781505033991 ) ) ;
#2003=CARTESIAN_POINT ( 'NONE',  ( -1.035533905932738197, -2.500000000000000000, -0.5430000000218496714 ) ) ;
#2007=CARTESIAN_POINT ( 'NONE',  ( 1.461580736456472573, 1.461580736456472795, 0.9500000010924747329 ) ) ;
#2011=CARTESIAN_POINT ( 'NONE',  ( -2.500000000000000444, 1.035533905932737753, 0.9500000021849498433 ) ) ;
#2022=CARTESIAN_POINT ( 'NONE',  ( 2.500000000000000444, 1.035533905932737975, -0.2500000000000002220 ) ) ;
#2023=PLANE ( 'NONE',  #12768 ) ;
#2029=( BOUNDED_CURVE ( )  B_SPLINE_CURVE ( 2, ( #2982, #4095, #13795, #5610, #10458, #4413, #6575, #14103, #2904 ),
 .UNSPECIFIED., .F., .F. ) 
 B_SPLINE_CURVE_WITH_KNOTS ( ( 3, 2, 2, 2, 3 ),
 ( 0.2142857142857142738, 0.2321428571428571508, 0.2500000000000000000, 0.2678571428571428492, 0.2857142857142856984 ),
 .UNSPECIFIED. ) 
 CURVE ( )  GEOMETRIC_REPRESENTATION_ITEM ( )  RATIONAL_B_SPLINE_CURVE ( ( 1.000000000000000000, 0.9238795325112867385, 1.000000000000000000, 0.9238795325112867385, 1.000000000000000000, 0.9238795325112867385, 1.000000000000000000, 0.9238795325112867385, 1.000000000000000000 ) ) 
 REPRESENTATION_ITEM ( '' )  );
#2031=CARTESIAN_POINT ( 'NONE',  ( -2.066987299999999195, -0.8561741729129467293, -1.899999998907525800 ) ) ;
#2050=ORIENTED_EDGE ( 'NONE', *, *, #201, .T. ) ;
#2060=CARTESIAN_POINT ( 'NONE',  ( -1.035533905932737753, 2.500000000000000444, 0.8500000021849498655 ) ) ;
#2064=CARTESIAN_POINT ( 'NONE',  ( 1.767766952966369320, -1.767766952966368654, 1.199999999999999956 ) ) ;
#2076=CARTESIAN_POINT ( 'NONE',  ( 1.767766952966369320, -1.767766952966368654, 1.300000002184949599 ) ) ;
#2080=CARTESIAN_POINT ( 'NONE',  ( 1.767766952966369320, -1.767766952966368654, 0.4069999999781502842 ) ) ;
#2086=FACE_OUTER_BOUND ( 'NONE', #6484, .T. ) ;
#2088=LINE ( 'NONE', #14505, #10875 ) ;
#2092=DIRECTION ( 'NONE',  ( 0.000000000000000000, 0.000000000000000000, -1.000000000000000000 ) ) ;
#2101=CARTESIAN_POINT ( 'NONE',  ( -1.767766952966369098, 1.767766952966369098, 0.000000000000000000 ) ) ;
#2125=DIRECTION ( 'NONE',  ( -1.000000000000000000, 0.000000000000000000, 0.000000000000000000 ) ) ;
#2135=DIRECTION ( 'NONE',  ( -0.4999999999999998890, 0.8660254037844387076, 0.000000000000000000 ) ) ;
#2136=CARTESIAN_POINT ( 'NONE',  ( -1.530808498934191571E-16, 2.500000000000000000, -1.599999997815050312 ) ) ;
#2139=CARTESIAN_POINT ( 'NONE',  ( -1.767766952966368432, -1.767766952966369320, 1.000000000000000000 ) ) ;
#2142=VECTOR ( 'NONE', #101, 1000.000000000000000 ) ;
#2144=ORIENTED_EDGE ( 'NONE', *, *, #12545, .F. ) ;
#2146=LINE ( 'NONE', #5085, #1906 ) ;
#2150=CARTESIAN_POINT ( 'NONE',  ( 3.796994071234844259E-16, -2.066987299999999639, 1.450000001092474733 ) ) ;
#2155=CARTESIAN_POINT ( 'NONE',  ( -1.035533905932737753, 2.500000000000000444, -0.04300000002184962283 ) ) ;
#2158=CARTESIAN_POINT ( 'NONE',  ( 0.8561741729129451750, 2.066987299999999639, 1.000000001092474555 ) ) ;
#2161=CARTESIAN_POINT ( 'NONE',  ( 1.035533905932737531, 2.500000000000000444, 0.7500000021849496656 ) ) ;
#2164=VECTOR ( 'NONE', #6272, 1000.000000000000000 ) ;
#2204=CARTESIAN_POINT ( 'NONE',  ( -1.265664690411614835E-16, 2.066987299999999639, -0.3499999989075254225 ) ) ;
#2217=CARTESIAN_POINT ( 'NONE',  ( 1.767766952966369320, -1.767766952966368654, 0.5000000021849496656 ) ) ;
#2221=CARTESIAN_POINT ( 'NONE',  ( 1.035533905932739085, -2.500000000000000000, 1.149999999999999689 ) ) ;
#2231=ADVANCED_FACE ( 'NONE', ( #10696 ), #987, .T. ) ;
#2232=CARTESIAN_POINT ( 'NONE',  ( 2.500000000000000444, 1.035533905932737975, -2.549999997815051156 ) ) ;
#2236=CARTESIAN_POINT ( 'NONE',  ( -2.500000000000000000, 0.000000000000000000, 0.1069999999781503230 ) ) ;
#2239=CARTESIAN_POINT ( 'NONE',  ( 2.066987299999999639, 2.531329380823229670E-16, -0.7499999989075251117 ) ) ;
#2257=DIRECTION ( 'NONE',  ( 0.000000000000000000, 0.000000000000000000, -1.000000000000000000 ) ) ;
#2277=CARTESIAN_POINT ( 'NONE',  ( 1.461580736456473018, -1.461580736456472573, 0.9500000010924747329 ) ) ;
#2285=CARTESIAN_POINT ( 'NONE',  ( 1.461580736456473018, -1.461580736456472573, 0.9500000010924747329 ) ) ;
#2299=CARTESIAN_POINT ( 'NONE',  ( 1.767766952966369320, -1.767766952966368654, 1.300000002184949821 ) ) ;
#2305=ORIENTED_EDGE ( 'NONE', *, *, #2400, .F. ) ;
#2312=CARTESIAN_POINT ( 'NONE',  ( 1.035533905932739085, -2.500000000000000000, -2.749999997815050445 ) ) ;
#2316=CARTESIAN_POINT ( 'NONE',  ( -1.530808498934191571E-16, 2.500000000000000000, -0.09300000002184975745 ) ) ;
#2318=CARTESIAN_POINT ( 'NONE',  ( -1.461580736456472351, -1.461580736456473018, 1.550000001092474822 ) ) ;
#2342=DIRECTION ( 'NONE',  ( 1.251928832280965695E-16, 1.000000000000000000, 0.000000000000000000 ) ) ;
#2356=CARTESIAN_POINT ( 'NONE',  ( 2.500000000000000000, 3.061616997868383141E-16, -0.1999999978150501789 ) ) ;
#2359=CARTESIAN_POINT ( 'NONE',  ( -1.461580736456472351, -1.461580736456473018, -0.04999999890752505893 ) ) ;
#2366=CARTESIAN_POINT ( 'NONE',  ( -0.8561741729129458411, -2.066987299999999195, -0.7999999989075252671 ) ) ;
#2367=CARTESIAN_POINT ( 'NONE',  ( -2.500000000000000000, 0.000000000000000000, 1.700000000000000178 ) ) ;
#2371=CARTESIAN_POINT ( 'NONE',  ( -2.500000000000000000, 0.000000000000000000, 1.800000002184949821 ) ) ;
#2381=CARTESIAN_POINT ( 'NONE',  ( 2.500000000000000000, 3.061616997868383141E-16, 0.5000000000000000000 ) ) ;
#2387=EDGE_CURVE ( 'NONE', #5765, #7968, #2736, .T. ) ;
#2390=ORIENTED_EDGE ( 'NONE', *, *, #771, .T. ) ;
#2393=CARTESIAN_POINT ( 'NONE',  ( -0.8561741729129455081, 2.066987299999999639, 1.900000001092474688 ) ) ;
#2397=CARTESIAN_POINT ( 'NONE',  ( -1.767766952966369098, 1.767766952966369098, 0.7999999999999999334 ) ) ;
#2400=EDGE_CURVE ( 'NONE', #7812, #1570, #4917, .T. ) ;
#2402=CARTESIAN_POINT ( 'NONE',  ( -0.8561741729129458411, -2.066987299999999195, -1.799999998907525267 ) ) ;
#2415=DIRECTION ( 'NONE',  ( 0.000000000000000000, 0.000000000000000000, -1.000000000000000000 ) ) ;
#2436=CARTESIAN_POINT ( 'NONE',  ( -2.283493650000000041, 0.000000000000000000, 1.925000001638712321 ) ) ;
#2440=CARTESIAN_POINT ( 'NONE',  ( 3.796994071234844259E-16, -2.066987299999999639, 1.650000001092474911 ) ) ;
#2447=CARTESIAN_POINT ( 'NONE',  ( -2.066987299999999639, 0.000000000000000000, 0.6500000010924747995 ) ) ;
#2449=CARTESIAN_POINT ( 'NONE',  ( -1.035533905932737753, 2.500000000000000444, 1.550000000000000266 ) ) ;
#2457=DIRECTION ( 'NONE',  ( 0.000000000000000000, 0.000000000000000000, -1.000000000000000000 ) ) ;
#2463=CARTESIAN_POINT ( 'NONE',  ( 4.592425496802573972E-16, -2.500000000000000000, -2.799999997815050268 ) ) ;
#2464=CARTESIAN_POINT ( 'NONE',  ( 0.000000000000000000, 0.000000000000000000, 2.500000000000000000 ) ) ;
#2475=VERTEX_POINT ( 'NONE', #3124 ) ;
#2478=CARTESIAN_POINT ( 'NONE',  ( 1.461580736456472573, 1.461580736456472795, 1.750000001092474999 ) ) ;
#2483=CARTESIAN_POINT ( 'NONE',  ( -1.035533905932737753, 2.500000000000000444, 2.350000000000000533 ) ) ;
#2487=CARTESIAN_POINT ( 'NONE',  ( -2.066987299999999639, 0.000000000000000000, 1.450000001092474955 ) ) ;
#2522=DIRECTION ( 'NONE',  ( 0.000000000000000000, 0.000000000000000000, 1.000000000000000000 ) ) ;
#2523=CARTESIAN_POINT ( 'NONE',  ( 2.066987299999999639, 2.531329380823229670E-16, 0.2500000010924748328 ) ) ;
#2530=CARTESIAN_POINT ( 'NONE',  ( 0.8561741729129452860, 2.066987299999999639, -0.3999999989075251339 ) ) ;
#2546=CARTESIAN_POINT ( 'NONE',  ( 2.500000000000000444, 1.035533905932737975, -2.549999997815051156 ) ) ;
#2553=( BOUNDED_CURVE ( )  B_SPLINE_CURVE ( 2, ( #13878, #2991, #6739, #1865, #9276, #10311, #14113, #6662, #5698 ),
 .UNSPECIFIED., .F., .F. ) 
 B_SPLINE_CURVE_WITH_KNOTS ( ( 3, 2, 2, 2, 3 ),
 ( 0.07142857142857142461, 0.08928571428571428770, 0.1071428571428571369, 0.1250000000000000000, 0.1428571428571428492 ),
 .UNSPECIFIED. ) 
 CURVE ( )  GEOMETRIC_REPRESENTATION_ITEM ( )  RATIONAL_B_SPLINE_CURVE ( ( 1.000000000000000000, 0.9238795325112867385, 1.000000000000000000, 0.9238795325112867385, 1.000000000000000000, 0.9238795325112867385, 1.000000000000000000, 0.9238795325112867385, 1.000000000000000000 ) ) 
 REPRESENTATION_ITEM ( '' )  );
#2558=CARTESIAN_POINT ( 'NONE',  ( 2.066987300000000083, -0.8561741729129449530, 0.8000000010924747107 ) ) ;
#2562=CARTESIAN_POINT ( 'NONE',  ( 4.592425496802573972E-16, -2.500000000000000000, 0.2999999999999999334 ) ) ;
#2565=CARTESIAN_POINT ( 'NONE',  ( 0.8561741729129451750, 2.066987299999999639, -1.399999998907525800 ) ) ;
#2571=CIRCLE ( 'NONE', #6652, 2.500000000000000000 ) ;
#2591=CARTESIAN_POINT ( 'NONE',  ( -1.035533905932737753, 2.500000000000000444, -0.8500000000000001998 ) ) ;
#2593=CARTESIAN_POINT ( 'NONE',  ( 0.000000000000000000, 0.000000000000000000, 2.500000000000000000 ) ) ;
#2595=CARTESIAN_POINT ( 'NONE',  ( 0.8561741729129451750, 2.066987299999999639, 2.000000001092475443 ) ) ;
#2602=CARTESIAN_POINT ( 'NONE',  ( 1.461580736456473018, -1.461580736456472573, -1.449999998907525178 ) ) ;
#2604=DIRECTION ( 'NONE',  ( 0.000000000000000000, 0.000000000000000000, -1.000000000000000000 ) ) ;
#2606=CARTESIAN_POINT ( 'NONE',  ( -1.461580736456472351, -1.461580736456473018, 0.5500000010924748217 ) ) ;
#2611=CARTESIAN_POINT ( 'NONE',  ( -1.500000000000000000, 0.000000000000000000, 2.500000000000000000 ) ) ;
#2621=CARTESIAN_POINT ( 'NONE',  ( 2.500000000000000444, -1.035533905932737309, -1.849999997815050090 ) ) ;
#2635=CARTESIAN_POINT ( 'NONE',  ( -0.8561741729129455081, 2.066987299999999639, -1.299999998907525267 ) ) ;
#2641=CARTESIAN_POINT ( 'NONE',  ( 2.500000000000000000, 3.061616997868383141E-16, 0.5000000000000000000 ) ) ;
#2646=CARTESIAN_POINT ( 'NONE',  ( -1.265664690411614835E-16, 2.066987299999999639, -2.949999998907525178 ) ) ;
#2667=ADVANCED_FACE ( 'NONE', ( #12258 ), #7262, .F. ) ;
#2676=CARTESIAN_POINT ( 'NONE',  ( -1.767766952966369098, 1.767766952966369098, 1.599999999999999867 ) ) ;
#2681=CARTESIAN_POINT ( 'NONE',  ( -1.767766952966368432, -1.767766952966369320, -2.099999997815050090 ) ) ;
#2683=CARTESIAN_POINT ( 'NONE',  ( -0.8561741729129458411, -2.066987299999999195, -1.599999998907525756 ) ) ;
#2699=CARTESIAN_POINT ( 'NONE',  ( -1.767766952966368432, -1.767766952966369320, -2.099999997815050090 ) ) ;
#2715=CARTESIAN_POINT ( 'NONE',  ( 2.066987300000000083, -0.8561741729129449530, -1.599999998907525534 ) ) ;
#2716=CARTESIAN_POINT ( 'NONE',  ( 2.500000000000000444, 1.035533905932737975, -1.850000000000000533 ) ) ;
#2719=CARTESIAN_POINT ( 'NONE',  ( 1.035533905932737531, 2.500000000000000444, 0.6500000000000000222 ) ) ;
#2723=CARTESIAN_POINT ( 'NONE',  ( 0.8561741729129451750, 2.066987299999999639, -0.3999999989075250784 ) ) ;
#2727=ORIENTED_EDGE ( 'NONE', *, *, #1242, .T. ) ;
#2736=LINE ( 'NONE', #14832, #3235 ) ;
#2757=CARTESIAN_POINT ( 'NONE',  ( 1.035533905932739085, -2.500000000000000000, 1.949999999999999956 ) ) ;
#2764=FACE_BOUND ( 'NONE', #5420, .T. ) ;
#2765=CARTESIAN_POINT ( 'NONE',  ( 1.767766984964215471, 1.767766920968521616, -2.500000000000000444 ) ) ;
#2766=CARTESIAN_POINT ( 'NONE',  ( -2.066987299999999639, 0.8561741729129455081, 1.200000001092474733 ) ) ;
#2786=EDGE_CURVE ( 'NONE', #1897, #12110, #1948, .T. ) ;
#2793=ORIENTED_EDGE ( 'NONE', *, *, #7772, .T. ) ;
#2794=CARTESIAN_POINT ( 'NONE',  ( 1.461580736456472573, 1.461580736456472795, -2.249999998907525001 ) ) ;
#2798=CARTESIAN_POINT ( 'NONE',  ( 2.500000000000000444, -1.035533905932737309, -0.3500000000000000333 ) ) ;
#2803=CARTESIAN_POINT ( 'NONE',  ( -0.8561741729129455081, 2.066987299999999639, -0.2999999989075253226 ) ) ;
#2808=VERTEX_POINT ( 'NONE', #11530 ) ;
#2810=EDGE_LOOP ( 'NONE', ( #11313, #12814, #9995, #6948 ) ) ;
#2839=CARTESIAN_POINT ( 'NONE',  ( -1.530808498934191571E-16, 2.500000000000000000, 2.299999999999999822 ) ) ;
#2846=CARTESIAN_POINT ( 'NONE',  ( -1.265664690411614835E-16, 2.066987299999999639, -1.949999998907525622 ) ) ;
#2852=ORIENTED_EDGE ( 'NONE', *, *, #11933, .T. ) ;
#2858=( BOUNDED_CURVE ( )  B_SPLINE_CURVE ( 2, ( #12059, #4751, #13488, #2591, #1390, #9770, #15572, #8581, #1084 ),
 .UNSPECIFIED., .F., .F. ) 
 B_SPLINE_CURVE_WITH_KNOTS ( ( 3, 2, 2, 2, 3 ),
 ( 0.5714285714285713969, 0.5892857142857143016, 0.6071428571428570953, 0.6250000000000000000, 0.6428571428571429047 ),
 .UNSPECIFIED. ) 
 CURVE ( )  GEOMETRIC_REPRESENTATION_ITEM ( )  RATIONAL_B_SPLINE_CURVE ( ( 1.000000000000000000, 0.9238795325112867385, 1.000000000000000000, 0.9238795325112867385, 1.000000000000000000, 0.9238795325112867385, 1.000000000000000000, 0.9238795325112867385, 1.000000000000000000 ) ) 
 REPRESENTATION_ITEM ( '' )  );
#2872=CARTESIAN_POINT ( 'NONE',  ( 0.8561741729129463963, -2.066987299999999195, -0.09999999890752520049 ) ) ;
#2876=CARTESIAN_POINT ( 'NONE',  ( -2.500000000000000444, 1.035533905932737753, -1.549999999999999600 ) ) ;
#2878=CARTESIAN_POINT ( 'NONE',  ( 2.500000000000000000, 3.061616997868383141E-16, -1.100000000000000311 ) ) ;
#2881=CARTESIAN_POINT ( 'NONE',  ( 2.066987299999999639, 2.531329380823229670E-16, 0.2500000010924748328 ) ) ;
#2896=CARTESIAN_POINT ( 'NONE',  ( 2.500000000000000444, 1.035533905932737975, 2.156999999978150395 ) ) ;
#2903=EDGE_LOOP ( 'NONE', ( #10669, #10071, #6382, #15255, #14376, #9527, #573, #9579, #11775, #14567, #8966, #5482, #1270, #11705, #7075 ) ) ;
#2904=CARTESIAN_POINT ( 'NONE',  ( -2.500000000000000000, 0.000000000000000000, 0.2000000021849497878 ) ) ;
#2905=ORIENTED_EDGE ( 'NONE', *, *, #12295, .T. ) ;
#2913=CARTESIAN_POINT ( 'NONE',  ( -1.035533905932738197, -2.500000000000000000, 1.849999999999999867 ) ) ;
#2915=( NAMED_UNIT ( * ) PLANE_ANGLE_UNIT ( ) SI_UNIT ( $, .RADIAN. ) );
#2924=CARTESIAN_POINT ( 'NONE',  ( 2.066987299999999639, 2.531329380823229670E-16, 1.650000001092474911 ) ) ;
#2945=ORIENTED_EDGE ( 'NONE', *, *, #4680, .F. ) ;
#2955=CARTESIAN_POINT ( 'NONE',  ( -1.767766952966369098, 1.767766952966369098, 1.700000002184949732 ) ) ;
#2959=CARTESIAN_POINT ( 'NONE',  ( -2.066987299999999639, 0.000000000000000000, -1.749999998907525223 ) ) ;
#2962=ORIENTED_EDGE ( 'NONE', *, *, #4651, .F. ) ;
#2964=ORIENTED_EDGE ( 'NONE', *, *, #11635, .T. ) ;
#2969=CARTESIAN_POINT ( 'NONE',  ( -1.767766952966369098, 1.767766952966369098, 1.700000002184949510 ) ) ;
#2982=CARTESIAN_POINT ( 'NONE',  ( 2.500000000000000000, 3.061616997868383141E-16, 0.6000000021849497545 ) ) ;
#2990=LINE ( 'NONE', #11185, #15292 ) ;
#2991=CARTESIAN_POINT ( 'NONE',  ( 2.500000000000000444, -1.035533905932737309, 2.050000000000000266 ) ) ;
#2992=CARTESIAN_POINT ( 'NONE',  ( -1.035533905932737753, 2.500000000000000444, -0.05000000000000014155 ) ) ;
#3001=CARTESIAN_POINT ( 'NONE',  ( -2.066987299999999639, 0.8561741729129455081, -0.3999999989075251339 ) ) ;
#3031=LINE ( 'NONE', #7961, #6429 ) ;
#3032=CARTESIAN_POINT ( 'NONE',  ( 1.035533905932737531, 2.500000000000000444, -0.1499999999999999667 ) ) ;
#3058=CARTESIAN_POINT ( 'NONE',  ( -1.224708070464005871, -2.198689805042928658, -2.500577006192093332 ) ) ;
#3068=CARTESIAN_POINT ( 'NONE',  ( -2.500000000000000444, 1.035533905932737753, 0.05000000000000014155 ) ) ;
#3070=CARTESIAN_POINT ( 'NONE',  ( 1.035533905932737531, 2.500000000000000444, 1.550000002184949821 ) ) ;
#3078=CARTESIAN_POINT ( 'NONE',  ( 2.066987300000000083, -0.8561741729129450640, -0.7999999989075252671 ) ) ;
#3095=CARTESIAN_POINT ( 'NONE',  ( 2.999999999999999556, 1.732050807568877859, -5.500000000000000000 ) ) ;
#3100=ORIENTED_EDGE ( 'NONE', *, *, #7862, .T. ) ;
#3108=CARTESIAN_POINT ( 'NONE',  ( -1.035533905932738197, -2.500000000000000000, -1.350000000000000089 ) ) ;
#3123=CARTESIAN_POINT ( 'NONE',  ( 1.035533905932737531, 2.500000000000000444, 0.7500000021849494436 ) ) ;
#3124=CARTESIAN_POINT ( 'NONE',  ( -2.500000000000000000, 0.000000000000000000, -2.199999997815050623 ) ) ;
#3128=CARTESIAN_POINT ( 'NONE',  ( 1.035533905932739085, -2.500000000000000000, 1.956999999978150662 ) ) ;
#3131=CARTESIAN_POINT ( 'NONE',  ( 1.461580736456472573, 1.461580736456472795, 1.750000001092474999 ) ) ;
#3137=CARTESIAN_POINT ( 'NONE',  ( 2.135184931484484849, 1.332301797266478571, -2.499207808506416661 ) ) ;
#3138=AXIS2_PLACEMENT_3D ( 'NONE', #12731, #11387, #10129 ) ;
#3146=CARTESIAN_POINT ( 'NONE',  ( 2.500000000000000444, -1.035533905932737309, -0.3500000000000000333 ) ) ;
#3155=CARTESIAN_POINT ( 'NONE',  ( -1.461580736456472351, -1.461580736456473018, -2.649999998907525356 ) ) ;
#3160=DIRECTION ( 'NONE',  ( 1.000000000000000000, 0.000000000000000000, 0.000000000000000000 ) ) ;
#3167=DIRECTION ( 'NONE',  ( 0.000000000000000000, 0.000000000000000000, -1.000000000000000000 ) ) ;
#3169=B_SPLINE_CURVE_WITH_KNOTS ( 'NONE', 3,
 ( #5541, #8080, #12839, #1942, #753, #3297 ),
 .UNSPECIFIED., .F., .F.,
 ( 4, 2, 4 ),
 ( 0.1250000000000000000, 0.1875000000000000000, 0.2500000000000000000 ),
 .UNSPECIFIED. ) ;
#3184=CARTESIAN_POINT ( 'NONE',  ( 1.035533905932739085, -2.500000000000000000, -0.3499999978150501456 ) ) ;
#3188=LINE ( 'NONE', #10353, #3417 ) ;
#3195=DIRECTION ( 'NONE',  ( 0.000000000000000000, 0.000000000000000000, -1.000000000000000000 ) ) ;
#3199=CARTESIAN_POINT ( 'NONE',  ( -2.500000000000000444, 1.035533905932737753, -0.6499999978150502455 ) ) ;
#3203=CARTESIAN_POINT ( 'NONE',  ( 1.767766952966368654, 1.767766952966369098, 1.406999999978150617 ) ) ;
#3205=CARTESIAN_POINT ( 'NONE',  ( -2.066987299999999195, -0.8561741729129466183, 0.5000000010924746663 ) ) ;
#3215=VERTEX_POINT ( 'NONE', #8101 ) ;
#3216=LINE ( 'NONE', #13072, #14785 ) ;
#3219=CARTESIAN_POINT ( 'NONE',  ( 1.035533905932737531, 2.500000000000000444, -0.9500000000000001776 ) ) ;
#3220=DIRECTION ( 'NONE',  ( 1.000000000000000000, -1.251928832280965695E-16, 0.000000000000000000 ) ) ;
#3221=SHAPE_REPRESENTATION_RELATIONSHIP ( 'NONE' , 'NONE' ,  #5305, #10501 ) ;
#3228=CARTESIAN_POINT ( 'NONE',  ( -1.461580736456472795, 1.461580736456472795, -0.4499999989075252338 ) ) ;
#3231=CARTESIAN_POINT ( 'NONE',  ( -2.500000000000000444, 1.035533905932737753, -1.449999997815050401 ) ) ;
#3235=VECTOR ( 'NONE', #187, 1000.000000000000227 ) ;
#3256=CARTESIAN_POINT ( 'NONE',  ( 1.767766952966369320, -1.767766952966368654, -0.2999999978150504343 ) ) ;
#3273=CARTESIAN_POINT ( 'NONE',  ( 4.592425496802573972E-16, -2.500000000000000000, -0.3999999978150504676 ) ) ;
#3278=CARTESIAN_POINT ( 'NONE',  ( -1.767766952966368432, -1.767766952966369320, -0.5930000000218498268 ) ) ;
#3280=ADVANCED_FACE ( 'NONE', ( #5716 ), #14315, .T. ) ;
#3283=CARTESIAN_POINT ( 'NONE',  ( -2.066987299999999639, 0.000000000000000000, -0.3499999989075254225 ) ) ;
#3291=CARTESIAN_POINT ( 'NONE',  ( -1.084202172485504434E-16, 3.464101615137754830, -2.500000000000000000 ) ) ;
#3297=CARTESIAN_POINT ( 'NONE',  ( -3.827021247335478803E-16, 2.500000000000000000, -2.500000000000000000 ) ) ;
#3299=CARTESIAN_POINT ( 'NONE',  ( -2.500000000000000000, -1.035533905932739307, 0.1499999999999999667 ) ) ;
#3300=DIRECTION ( 'NONE',  ( 0.8660254037844385966, -0.4999999999999998890, 0.000000000000000000 ) ) ;
#3309=CARTESIAN_POINT ( 'NONE',  ( 0.8561741729129452860, 2.066987299999999639, -1.399999998907526022 ) ) ;
#3310=PRODUCT_DEFINITION ( 'UNKNOWN', '', #4265, #6590 ) ;
#3315=ORIENTED_EDGE ( 'NONE', *, *, #1976, .T. ) ;
#3319=CARTESIAN_POINT ( 'NONE',  ( -1.530808498934191571E-16, 2.500000000000000000, -3.199999997815050623 ) ) ;
#3325=CARTESIAN_POINT ( 'NONE',  ( -2.500000000000000000, -1.035533905932739307, 1.050000002184949821 ) ) ;
#3335=CARTESIAN_POINT ( 'NONE',  ( 1.767766952966368654, 1.767766952966369098, -0.09999999781505011787 ) ) ;
#3339=CARTESIAN_POINT ( 'NONE',  ( 1.461580736456473018, -1.461580736456472573, -2.249999998907525445 ) ) ;
#3350=CARTESIAN_POINT ( 'NONE',  ( 1.035533905932737531, 2.500000000000000444, -2.449999997815050179 ) ) ;
#3354=CARTESIAN_POINT ( 'NONE',  ( -2.500000000000000000, -1.035533905932739307, -0.6430000000218495382 ) ) ;
#3356=CARTESIAN_POINT ( 'NONE',  ( -0.8561741729129455081, 2.066987299999999639, 1.100000001092475088 ) ) ;
#3360=CARTESIAN_POINT ( 'NONE',  ( 2.500000000000000444, 1.035533905932737975, 0.6500000021849499099 ) ) ;
#3362=DIRECTION ( 'NONE',  ( 0.000000000000000000, 0.000000000000000000, 1.000000000000000000 ) ) ;
#3369=EDGE_LOOP ( 'NONE', ( #14239, #7079, #9, #6960 ) ) ;
#3385=VERTEX_POINT ( 'NONE', #5429 ) ;
#3389=CIRCLE ( 'NONE', #4933, 1.500000000000000222 ) ;
#3396=EDGE_CURVE ( 'NONE', #10225, #1897, #13336, .T. ) ;
#3397=CYLINDRICAL_SURFACE ( 'NONE', #5473, 2.500000000000000000 ) ;
#3398=CARTESIAN_POINT ( 'NONE',  ( 3.796994071234844259E-16, -2.066987299999999639, -0.7499999989075251117 ) ) ;
#3407=CARTESIAN_POINT ( 'NONE',  ( -1.767766952966369098, 1.767766952966369098, 0.1000000021849497545 ) ) ;
#3411=CARTESIAN_POINT ( 'NONE',  ( -1.767766952966369098, 1.767766952966369098, -0.6999999978150501789 ) ) ;
#3412=CARTESIAN_POINT ( 'NONE',  ( 0.000000000000000000, 0.000000000000000000, 2.500000000000000000 ) ) ;
#3417=VECTOR ( 'NONE', #564, 1000.000000000000000 ) ;
#3419=ORIENTED_EDGE ( 'NONE', *, *, #5808, .F. ) ;
#3424=CARTESIAN_POINT ( 'NONE',  ( 4.592425496802573972E-16, -2.500000000000000000, -1.999999997815050445 ) ) ;
#3430=CARTESIAN_POINT ( 'NONE',  ( -2.500000000000000000, 0.000000000000000000, -1.493000000021849516 ) ) ;
#3433=CARTESIAN_POINT ( 'NONE',  ( 2.066987299999999639, 0.8561741729129456191, -0.6999999989075255113 ) ) ;
#3434=CARTESIAN_POINT ( 'NONE',  ( -1.767766952966369098, 1.767766952966369098, -2.399999999999999911 ) ) ;
#3437=VERTEX_POINT ( 'NONE', #715 ) ;
#3442=EDGE_LOOP ( 'NONE', ( #5747, #15057, #6342, #8924, #3756, #8560, #12034, #14309, #801, #10670, #13109, #3467, #10485, #15607, #941, #11951 ) ) ;
#3451=CARTESIAN_POINT ( 'NONE',  ( 2.500000000000000444, -1.035533905932737309, -1.049999997815050268 ) ) ;
#3452=( BOUNDED_CURVE ( )  B_SPLINE_CURVE ( 2, ( #4210, #1813, #6685, #10803, #4925, #58, #7234, #9780, #9537, #15584, #933, #10645, #13344, #12151, #14626, #1096, #12073, #8349, #3638, #13188, #4686, #8513, #14374, #11991, #3479, #5880, #2285, #3715, #14461, #7073, #9702, #8592, #2447, #15507, #13104, #6126, #4605, #13426, #1250, #7311, #10961, #5959, #7154, #3562, #9622, #9456, #15663, #4764, #1171, #8430, #5799, #10885, #2204, #2530, #10726, #11909, #7385, #6040, #13267, #14291, #3398, #2366, #8267, #6808, #4847, #14540, #1017, #3945, #14858, #136, #7535, #3868, #8903, #372, #2602, #10011, #8819, #2683, #9854, #12542, #9931, #13738, #6359, #220, #2846, #1481, #5240, #1639, #5156, #14782, #13574, #12462, #12382, #7617, #14703, #5001, #10164, #6440, #13649, #1326, #8981 ),
 .UNSPECIFIED., .F., .F. ) 
 B_SPLINE_CURVE_WITH_KNOTS ( ( 3, 2, 2, 2, 2, 2, 2, 2, 2, 2, 2, 2, 2, 2, 2, 2, 2, 2, 2, 2, 2, 2, 2, 2, 2, 2, 2, 2, 2, 2, 2, 2, 2, 2, 2, 2, 2, 2, 2, 2, 2, 2, 2, 2, 2, 2, 2, 2, 2, 2, 3 ),
 ( 0.000000000000000000, 0.01785714285714285615, 0.03571428571428571230, 0.05357142857142856845, 0.07142857142857142461, 0.08928571428571428770, 0.1071428571428571369, 0.1250000000000000000, 0.1428571428571428492, 0.1607142857142857262, 0.1785714285714285754, 0.1964285714285714246, 0.2142857142857142738, 0.2321428571428571508, 0.2500000000000000000, 0.2678571428571428492, 0.2857142857142856984, 0.3035714285714285476, 0.3214285714285714524, 0.3392857142857143016, 0.3571428571428571508, 0.3750000000000000000, 0.3928571428571428492, 0.4107142857142856984, 0.4285714285714285476, 0.4464285714285714524, 0.4642857142857143016, 0.4821428571428571508, 0.5000000000000000000, 0.5178571428571429047, 0.5357142857142856984, 0.5535714285714286031, 0.5714285714285713969, 0.5892857142857143016, 0.6071428571428570953, 0.6250000000000000000, 0.6428571428571429047, 0.6607142857142856984, 0.6785714285714286031, 0.6964285714285715079, 0.7142857142857143016, 0.7321428571428570953, 0.7500000000000000000, 0.7678571428571429047, 0.7857142857142856984, 0.8035714285714286031, 0.8214285714285713969, 0.8392857142857143016, 0.8571428571428570953, 0.8750000000000000000, 0.8928571428571429047 ),
 .UNSPECIFIED. ) 
 CURVE ( )  GEOMETRIC_REPRESENTATION_ITEM ( )  RATIONAL_B_SPLINE_CURVE ( ( 1.000000000000000000, 0.9238795325112867385, 1.000000000000000000, 0.9238795325112867385, 1.000000000000000000, 0.9238795325112867385, 1.000000000000000000, 0.9238795325112867385, 1.000000000000000000, 0.9238795325112867385, 1.000000000000000000, 0.9238795325112867385, 1.000000000000000000, 0.9238795325112867385, 1.000000000000000000, 0.9238795325112867385, 1.000000000000000000, 0.9238795325112867385, 1.000000000000000000, 0.9238795325112867385, 1.000000000000000000, 0.9238795325112867385, 1.000000000000000000, 0.9238795325112867385, 1.000000000000000000, 0.9238795325112867385, 1.000000000000000000, 0.9238795325112867385, 1.000000000000000000, 0.9238795325112867385, 1.000000000000000000, 0.9238795325112867385, 1.000000000000000000, 0.9238795325112867385, 1.000000000000000000, 0.9238795325112867385, 1.000000000000000000, 0.9238795325112867385, 1.000000000000000000, 0.9238795325112867385, 1.000000000000000000, 0.9238795325112867385, 1.000000000000000000, 0.9238795325112867385, 1.000000000000000000, 0.9238795325112867385, 1.000000000000000000, 0.9238795325112867385, 1.000000000000000000, 0.9238795325112867385, 1.000000000000000000, 0.9238795325112867385, 1.000000000000000000, 0.9238795325112867385, 1.000000000000000000, 0.9238795325112867385, 1.000000000000000000, 0.9238795325112867385, 1.000000000000000000, 0.9238795325112867385, 1.000000000000000000, 0.9238795325112867385, 1.000000000000000000, 0.9238795325112867385, 1.000000000000000000, 0.9238795325112867385, 1.000000000000000000, 0.9238795325112867385, 1.000000000000000000, 0.9238795325112867385, 1.000000000000000000, 0.9238795325112867385, 1.000000000000000000, 0.9238795325112867385, 1.000000000000000000, 0.9238795325112867385, 1.000000000000000000, 0.9238795325112867385, 1.000000000000000000, 0.9238795325112867385, 1.000000000000000000, 0.9238795325112867385, 1.000000000000000000, 0.9238795325112867385, 1.000000000000000000, 0.9238795325112867385, 1.000000000000000000, 0.9238795325112867385, 1.000000000000000000, 0.9238795325112867385, 1.000000000000000000, 0.9238795325112867385, 1.000000000000000000, 0.9238795325112867385, 1.000000000000000000, 0.9238795325112867385, 1.000000000000000000, 0.9238795325112867385, 1.000000000000000000, 0.9238795325112867385, 1.000000000000000000 ) ) 
 REPRESENTATION_ITEM ( '' )  );
#3458=EDGE_CURVE ( 'NONE', #8784, #15622, #209, .T. ) ;
#3464=DIRECTION ( 'NONE',  ( -1.000000000000000000, 0.000000000000000000, 0.000000000000000000 ) ) ;
#3467=ORIENTED_EDGE ( 'NONE', *, *, #2786, .T. ) ;
#3470=CARTESIAN_POINT ( 'NONE',  ( -2.500000000000000000, 0.000000000000000000, -0.5999999978150503122 ) ) ;
#3471=CARTESIAN_POINT ( 'NONE',  ( 2.066987299999999639, 0.8561741729129456191, -0.4999999989075253337 ) ) ;
#3479=CARTESIAN_POINT ( 'NONE',  ( 2.066987299999999639, 2.531329380823229670E-16, 1.050000001092474822 ) ) ;
#3481=ORIENTED_EDGE ( 'NONE', *, *, #2786, .F. ) ;
#3495=CARTESIAN_POINT ( 'NONE',  ( -2.500000000000000000, 0.000000000000000000, 0.2000000021849497878 ) ) ;
#3497=LINE ( 'NONE', #12088, #6196 ) ;
#3499=CARTESIAN_POINT ( 'NONE',  ( -2.500000000000000000, 0.000000000000000000, 0.9000000000000000222 ) ) ;
#3511=CARTESIAN_POINT ( 'NONE',  ( 0.8561741729129451750, 2.066987299999999639, 1.800000001092475266 ) ) ;
#3515=CARTESIAN_POINT ( 'NONE',  ( -1.035533905932738197, -2.500000000000000000, 1.056999999978150528 ) ) ;
#3518=CARTESIAN_POINT ( 'NONE',  ( -1.265664690411614835E-16, 2.066987299999999639, 2.050000001092474822 ) ) ;
#3530=DIRECTION ( 'NONE',  ( -0.8660254037844385966, 0.5000000000000001110, 0.000000000000000000 ) ) ;
#3554=CARTESIAN_POINT ( 'NONE',  ( -0.8561741729129455081, 2.066987299999999639, 2.100000001092475088 ) ) ;
#3562=CARTESIAN_POINT ( 'NONE',  ( 0.8561741729129465073, -2.066987299999999195, 0.1000000010924748939 ) ) ;
#3574=PLANE ( 'NONE',  #11992 ) ;
#3575=CARTESIAN_POINT ( 'NONE',  ( 4.592425496802573972E-16, -2.500000000000000000, -1.999999997815050001 ) ) ;
#3578=CARTESIAN_POINT ( 'NONE',  ( -1.035533905932738197, -2.500000000000000000, 1.050000000000000044 ) ) ;
#3580=( BOUNDED_CURVE ( )  B_SPLINE_CURVE ( 2, ( #7231, #12069, #12379, #8739, #3866, #1636, #8665, #7456, #11557 ),
 .UNSPECIFIED., .F., .F. ) 
 B_SPLINE_CURVE_WITH_KNOTS ( ( 3, 2, 2, 2, 3 ),
 ( 0.5000000000000000000, 0.5178571428571429047, 0.5357142857142856984, 0.5535714285714286031, 0.5714285714285713969 ),
 .UNSPECIFIED. ) 
 CURVE ( )  GEOMETRIC_REPRESENTATION_ITEM ( )  RATIONAL_B_SPLINE_CURVE ( ( 1.000000000000000000, 0.9238795325112867385, 1.000000000000000000, 0.9238795325112867385, 1.000000000000000000, 0.9238795325112867385, 1.000000000000000000, 0.9238795325112867385, 1.000000000000000000 ) ) 
 REPRESENTATION_ITEM ( '' )  );
#3582=EDGE_LOOP ( 'NONE', ( #15288, #2852, #6086, #12405 ) ) ;
#3588=CARTESIAN_POINT ( 'NONE',  ( -1.767766952966369098, 1.767766952966369098, -1.499999997815050223 ) ) ;
#3593=CARTESIAN_POINT ( 'NONE',  ( 2.500000000000000444, 1.035533905932737975, -1.843000000021850049 ) ) ;
#3595=CARTESIAN_POINT ( 'NONE',  ( 2.066987300000000083, -0.8561741729129449530, 1.800000001092475266 ) ) ;
#3601=EDGE_LOOP ( 'NONE', ( #11081, #180, #8706, #9195 ) ) ;
#3602=CYLINDRICAL_SURFACE ( 'NONE', #13654, 2.500000000000000000 ) ;
#3611=ADVANCED_FACE ( 'NONE', ( #9391 ), #14303, .F. ) ;
#3631=CARTESIAN_POINT ( 'NONE',  ( 2.066987300000000083, -0.8561741729129449530, 1.800000001092475266 ) ) ;
#3638=CARTESIAN_POINT ( 'NONE',  ( -1.461580736456472795, 1.461580736456472795, 1.350000001092474644 ) ) ;
#3651=CARTESIAN_POINT ( 'NONE',  ( 2.999999999999999556, -1.732050807568877859, -5.500000000000000000 ) ) ;
#3652=CARTESIAN_POINT ( 'NONE',  ( 1.767766952966368654, 1.767766952966369098, -2.499999997815050445 ) ) ;
#3667=CARTESIAN_POINT ( 'NONE',  ( -1.767766952966369098, 1.767766952966369098, -2.299999997815050712 ) ) ;
#3669=CARTESIAN_POINT ( 'NONE',  ( 1.035533905932737531, 2.500000000000000444, -0.1499999999999999944 ) ) ;
#3671=CARTESIAN_POINT ( 'NONE',  ( -2.500000000000000000, -0.4783542904563624076, 2.523096988312782063 ) ) ;
#3675=CARTESIAN_POINT ( 'NONE',  ( -2.066987299999999639, 0.8561741729129452860, -2.799999998907525267 ) ) ;
#3676=CARTESIAN_POINT ( 'NONE',  ( -2.500000000000000000, 0.000000000000000000, -2.300000000000000266 ) ) ;
#3681=ORIENTED_EDGE ( 'NONE', *, *, #1143, .T. ) ;
#3691=CARTESIAN_POINT ( 'NONE',  ( -2.500000000000000000, 0.000000000000000000, -2.300000000000000266 ) ) ;
#3699=EDGE_CURVE ( 'NONE', #786, #4232, #1417, .T. ) ;
#3708=CARTESIAN_POINT ( 'NONE',  ( -1.265664690411614835E-16, 2.066987299999999639, 0.4500000010924747329 ) ) ;
#3715=CARTESIAN_POINT ( 'NONE',  ( 0.8561741729129465073, -2.066987299999999195, 0.9000000010924746885 ) ) ;
#3724=FILL_AREA_STYLE ('',( #5967 ) ) ;
#3741=DIRECTION ( 'NONE',  ( 0.000000000000000000, 0.000000000000000000, -1.000000000000000000 ) ) ;
#3743=CARTESIAN_POINT ( 'NONE',  ( -2.066987299999999195, -0.8561741729129466183, 0.5000000010924746663 ) ) ;
#3744=DIRECTION ( 'NONE',  ( 0.8660254037844385966, -0.4999999999999999445, 0.000000000000000000 ) ) ;
#3748=CARTESIAN_POINT ( 'NONE',  ( 1.767766952966368654, 1.767766952966369098, 0.6000000000000000888 ) ) ;
#3753=CARTESIAN_POINT ( 'NONE',  ( -2.066987299999999639, 0.8561741729129452860, -1.199999998907525622 ) ) ;
#3756=ORIENTED_EDGE ( 'NONE', *, *, #11823, .T. ) ;
#3769=CARTESIAN_POINT ( 'NONE',  ( 2.500000000000000000, 3.061616997868383141E-16, 2.100000000000000089 ) ) ;
#3772=AXIS2_PLACEMENT_3D ( 'NONE', #4315, #3195, #11544 ) ;
#3781=DIRECTION ( 'NONE',  ( 0.000000000000000000, 0.000000000000000000, 1.000000000000000000 ) ) ;
#3783=LINE ( 'NONE', #10876, #4627 ) ;
#3784=CARTESIAN_POINT ( 'NONE',  ( -1.265664690411614835E-16, 2.066987299999999639, -0.3499999989075254225 ) ) ;
#3789=DIRECTION ( 'NONE',  ( 0.000000000000000000, -1.000000000000000000, 0.000000000000000000 ) ) ;
#3792=DIRECTION ( 'NONE',  ( -1.000000000000000000, 0.000000000000000000, 0.000000000000000000 ) ) ;
#3796=CARTESIAN_POINT ( 'NONE',  ( -0.8561741729129458411, -2.066987299999999195, 0.6000000010924746441 ) ) ;
#3799=DIRECTION ( 'NONE',  ( 6.123233995736782060E-17, -1.000000000000000000, 0.000000000000000000 ) ) ;
#3801=VERTEX_POINT ( 'NONE', #7249 ) ;
#3803=DIRECTION ( 'NONE',  ( 0.000000000000000000, 0.000000000000000000, -1.000000000000000000 ) ) ;
#3821=FACE_OUTER_BOUND ( 'NONE', #3369, .T. ) ;
#3823=CARTESIAN_POINT ( 'NONE',  ( -2.066987299999999639, 0.000000000000000000, -0.3499999989075254225 ) ) ;
#3827=CARTESIAN_POINT ( 'NONE',  ( -1.530808498934191571E-16, 2.500000000000000000, 1.500000000000000000 ) ) ;
#3829=EDGE_CURVE ( 'NONE', #8784, #6636, #15711, .T. ) ;
#3831=CARTESIAN_POINT ( 'NONE',  ( -2.066987299999999639, 0.000000000000000000, -2.749999998907525445 ) ) ;
#3837=AXIS2_PLACEMENT_3D ( 'NONE', #2593, #12062, #49 ) ;
#3852=CARTESIAN_POINT ( 'NONE',  ( -3.827021247335478803E-16, 2.500000000000000000, -2.500000000000000000 ) ) ;
#3862=CARTESIAN_POINT ( 'NONE',  ( -0.8561741729129458411, -2.066987299999999195, -1.599999998907525534 ) ) ;
#3866=CARTESIAN_POINT ( 'NONE',  ( 4.592425496802573972E-16, -2.500000000000000000, -0.5000000000000000000 ) ) ;
#3868=CARTESIAN_POINT ( 'NONE',  ( 2.066987299999999639, 0.8561741729129456191, -1.299999998907525267 ) ) ;
#3869=CARTESIAN_POINT ( 'NONE',  ( 4.592425496802573972E-16, -2.500000000000000000, -2.799999997815050268 ) ) ;
#3871=CARTESIAN_POINT ( 'NONE',  ( 2.066987299999999639, 2.531329380823229670E-16, 0.8500000010924746441 ) ) ;
#3876=CARTESIAN_POINT ( 'NONE',  ( 0.000000000000000000, 0.000000000000000000, 2.500000000000000000 ) ) ;
#3897=CARTESIAN_POINT ( 'NONE',  ( 2.066987299999999639, 0.8561741729129456191, -1.499999998907525445 ) ) ;
#3902=CARTESIAN_POINT ( 'NONE',  ( -2.500000000000000000, -1.035533905932739307, -2.243000000021849516 ) ) ;
#3906=CARTESIAN_POINT ( 'NONE',  ( 2.066987300000000083, -0.8561741729129449530, 0.2000000010924747329 ) ) ;
#3937=CARTESIAN_POINT ( 'NONE',  ( 2.066987299999999639, 2.531329380823229670E-16, -2.149999998907525356 ) ) ;
#3942=CARTESIAN_POINT ( 'NONE',  ( 4.592425496802573972E-16, -2.500000000000000000, -1.999999997815050001 ) ) ;
#3945=CARTESIAN_POINT ( 'NONE',  ( -0.8561741729129455081, 2.066987299999999639, -1.099999998907525312 ) ) ;
#3948=CARTESIAN_POINT ( 'NONE',  ( 1.461580736456472573, 1.461580736456472795, 1.750000001092474999 ) ) ;
#3975=CARTESIAN_POINT ( 'NONE',  ( 1.461580736456473018, -1.461580736456472573, -0.04999999890752549608 ) ) ;
#3976=CARTESIAN_POINT ( 'NONE',  ( 1.767766952966368654, 1.767766952966369098, -1.800000000000000044 ) ) ;
#3979=CARTESIAN_POINT ( 'NONE',  ( -1.767766952966369098, 1.767766952966369098, -1.600000000000000311 ) ) ;
#3982=CARTESIAN_POINT ( 'NONE',  ( -0.8561741729129458411, -2.066987299999999195, 0.8000000010924747107 ) ) ;
#4020=CARTESIAN_POINT ( 'NONE',  ( 3.796994071234844259E-16, -2.066987299999999639, -1.549999998907525045 ) ) ;
#4029=CARTESIAN_POINT ( 'NONE',  ( -2.066987299999999639, 0.000000000000000000, 1.250000001092474777 ) ) ;
#4041=DIRECTION ( 'NONE',  ( 1.000000000000000000, 0.000000000000000000, 0.000000000000000000 ) ) ;
#4059=ORIENTED_EDGE ( 'NONE', *, *, #6920, .T. ) ;
#4060=CARTESIAN_POINT ( 'NONE',  ( 2.066987299999999639, 2.531329380823229670E-16, -1.549999998907525489 ) ) ;
#4064=CARTESIAN_POINT ( 'NONE',  ( -2.500000000000000444, 1.035533905932737753, -0.7500000000000004441 ) ) ;
#4069=CARTESIAN_POINT ( 'NONE',  ( -2.066987299999999639, 0.000000000000000000, -0.9499999989075252893 ) ) ;
#4085=CARTESIAN_POINT ( 'NONE',  ( -1.767766952966369098, 1.767766952966369098, 1.606999999978150351 ) ) ;
#4095=CARTESIAN_POINT ( 'NONE',  ( 2.500000000000000444, -1.035533905932737309, 0.5500000021849498211 ) ) ;
#4105=CARTESIAN_POINT ( 'NONE',  ( 1.461580736456473018, -1.461580736456472573, -1.449999998907525178 ) ) ;
#4112=CARTESIAN_POINT ( 'NONE',  ( 1.767766952966369320, -1.767766952966368654, -2.699999997815051067 ) ) ;
#4113=CARTESIAN_POINT ( 'NONE',  ( 1.461580736456472573, 1.461580736456472795, 0.9500000010924747329 ) ) ;
#4134=ORIENTED_EDGE ( 'NONE', *, *, #4680, .T. ) ;
#4137=ORIENTED_EDGE ( 'NONE', *, *, #14948, .F. ) ;
#4139=CARTESIAN_POINT ( 'NONE',  ( -2.500000000000000000, 0.000000000000000000, -1.500000000000000000 ) ) ;
#4141=CARTESIAN_POINT ( 'NONE',  ( 0.4831378333609244180, 2.500000000000000000, -2.523327958195909826 ) ) ;
#4147=CARTESIAN_POINT ( 'NONE',  ( 2.066987299999999639, 0.8561741729129456191, 1.100000001092475088 ) ) ;
#4159=AXIS2_PLACEMENT_3D ( 'NONE', #10804, #14463, #7235 ) ;
#4172=( BOUNDED_CURVE ( )  B_SPLINE_CURVE ( 2, ( #9676, #3451, #6970, #8319, #7128, #7207, #13158, #11803, #10621 ),
 .UNSPECIFIED., .F., .F. ) 
 B_SPLINE_CURVE_WITH_KNOTS ( ( 3, 2, 2, 2, 3 ),
 ( 0.5000000000000000000, 0.5178571428571429047, 0.5357142857142856984, 0.5535714285714286031, 0.5714285714285713969 ),
 .UNSPECIFIED. ) 
 CURVE ( )  GEOMETRIC_REPRESENTATION_ITEM ( )  RATIONAL_B_SPLINE_CURVE ( ( 1.000000000000000000, 0.9238795325112867385, 1.000000000000000000, 0.9238795325112867385, 1.000000000000000000, 0.9238795325112867385, 1.000000000000000000, 0.9238795325112867385, 1.000000000000000000 ) ) 
 REPRESENTATION_ITEM ( '' )  );
#4183=CARTESIAN_POINT ( 'NONE',  ( 0.8561741729129463963, -2.066987299999999195, -1.499999998907525445 ) ) ;
#4193=CARTESIAN_POINT ( 'NONE',  ( -0.8561741729129458411, -2.066987299999999195, -0.1999999989075254836 ) ) ;
#4210=CARTESIAN_POINT ( 'NONE',  ( -2.066987299999999639, 0.000000000000000000, 2.250000001092474999 ) ) ;
#4219=CARTESIAN_POINT ( 'NONE',  ( -0.8561741729129455081, 2.066987299999999639, -2.899999998907526244 ) ) ;
#4222=CARTESIAN_POINT ( 'NONE',  ( 1.767766952966369320, -1.767766952966368654, -2.000000000000000444 ) ) ;
#4226=CARTESIAN_POINT ( 'NONE',  ( 1.461580736456472573, 1.461580736456472795, -1.249999998907525223 ) ) ;
#4232=VERTEX_POINT ( 'NONE', #14414 ) ;
#4238=CARTESIAN_POINT ( 'NONE',  ( 2.500000000000000444, 1.035533905932737975, -0.1499999978150504398 ) ) ;
#4250=CARTESIAN_POINT ( 'NONE',  ( -0.4013174258278009998, -2.483589256803624412, -2.498872199792083304 ) ) ;
#4262=CARTESIAN_POINT ( 'NONE',  ( -1.767766952966369098, 1.767766952966369098, -0.7999999999999999334 ) ) ;
#4265=PRODUCT_DEFINITION_FORMATION_WITH_SPECIFIED_SOURCE ( 'ANY', '', #6017, .NOT_KNOWN. ) ;
#4271=CARTESIAN_POINT ( 'NONE',  ( 2.066987299999999639, 0.8561741729129456191, -1.499999998907525445 ) ) ;
#4275=CARTESIAN_POINT ( 'NONE',  ( 1.035533905932737531, 2.500000000000000444, -1.649999997815050579 ) ) ;
#4277=CARTESIAN_POINT ( 'NONE',  ( -3.827021247335478803E-16, 2.500000000000000000, -2.500000000000000000 ) ) ;
#4301=EDGE_CURVE ( 'NONE', #11794, #13528, #836, .T. ) ;
#4303=CARTESIAN_POINT ( 'NONE',  ( 1.767766952966368654, 1.767766952966369098, -1.800000000000000044 ) ) ;
#4315=CARTESIAN_POINT ( 'NONE',  ( 0.000000000000000000, 0.000000000000000000, -5.500000000000000000 ) ) ;
#4317=CARTESIAN_POINT ( 'NONE',  ( -2.500000000000000000, -1.035533905932739307, 0.2500000021849494991 ) ) ;
#4323=CARTESIAN_POINT ( 'NONE',  ( 1.035533905932737531, 2.500000000000000444, 2.256999999978151372 ) ) ;
#4327=CARTESIAN_POINT ( 'NONE',  ( -2.066987299999999639, 0.8561741729129452860, 1.200000001092474733 ) ) ;
#4333=CARTESIAN_POINT ( 'NONE',  ( 2.502037656352691375, 0.09969062346262420882, -2.500435595467218164 ) ) ;
#4342=CARTESIAN_POINT ( 'NONE',  ( -1.767766952966368432, -1.767766952966369320, -0.6000000000000003109 ) ) ;
#4352=CARTESIAN_POINT ( 'NONE',  ( 3.796994071234844259E-16, -2.066987299999999639, -2.549999998907525267 ) ) ;
#4355=CARTESIAN_POINT ( 'NONE',  ( 2.500000000000000444, 1.035533905932737975, -1.749999997815050445 ) ) ;
#4385=CARTESIAN_POINT ( 'NONE',  ( -1.767766952966368432, -1.767766952966369320, 1.100000002184950088 ) ) ;
#4400=CARTESIAN_POINT ( 'NONE',  ( 1.035533905932737531, 2.500000000000000444, 1.550000002184949599 ) ) ;
#4405=CARTESIAN_POINT ( 'NONE',  ( 1.035533905932737531, 2.500000000000000444, 1.456999999978150662 ) ) ;
#4408=CARTESIAN_POINT ( 'NONE',  ( 2.066987299999999639, 0.8561741729129456191, 0.1000000010924746996 ) ) ;
#4413=CARTESIAN_POINT ( 'NONE',  ( -1.035533905932738197, -2.500000000000000000, 0.3500000021849497545 ) ) ;
#4420=LINE ( 'NONE', #1941, #12725 ) ;
#4422=CARTESIAN_POINT ( 'NONE',  ( 1.767766952966369320, -1.767766952966368654, 0.3999999999999997446 ) ) ;
#4429=CARTESIAN_POINT ( 'NONE',  ( -1.461580736456472795, 1.461580736456472795, -2.849999998907525089 ) ) ;
#4432=DIRECTION ( 'NONE',  ( -1.000000000000000000, 0.000000000000000000, 0.000000000000000000 ) ) ;
#4458=CARTESIAN_POINT ( 'NONE',  ( -1.767766952966369098, 1.767766952966369098, 0.9000000021849497989 ) ) ;
#4462=CARTESIAN_POINT ( 'NONE',  ( 2.500000000000000444, -1.035533905932737309, 1.250000000000000222 ) ) ;
#4468=ORIENTED_EDGE ( 'NONE', *, *, #6435, .F. ) ;
#4472=CARTESIAN_POINT ( 'NONE',  ( -1.767766952966368432, -1.767766952966369320, -0.4999999978150503344 ) ) ;
#4477=CARTESIAN_POINT ( 'NONE',  ( -1.035533905932738197, -2.500000000000000000, 0.2569999999781503175 ) ) ;
#4480=CARTESIAN_POINT ( 'NONE',  ( 0.8561741729129463963, -2.066987299999999195, -0.09999999890752520049 ) ) ;
#4492=VERTEX_POINT ( 'NONE', #360 ) ;
#4497=CARTESIAN_POINT ( 'NONE',  ( -2.500000000000000000, 0.000000000000000000, -1.500000000000000000 ) ) ;
#4506=CARTESIAN_POINT ( 'NONE',  ( -1.461580736456472351, -1.461580736456473018, -1.049999998907525489 ) ) ;
#4509=FACE_OUTER_BOUND ( 'NONE', #2810, .T. ) ;
#4517=CARTESIAN_POINT ( 'NONE',  ( -2.500000000000000000, -1.035533905932739307, -0.5499999978150503788 ) ) ;
#4524=DIRECTION ( 'NONE',  ( 0.000000000000000000, 0.000000000000000000, 1.000000000000000000 ) ) ;
#4535=DIRECTION ( 'NONE',  ( 0.000000000000000000, 0.000000000000000000, -1.000000000000000000 ) ) ;
#4540=CARTESIAN_POINT ( 'NONE',  ( -1.035533905932738197, -2.500000000000000000, -1.249999997815050223 ) ) ;
#4543=CARTESIAN_POINT ( 'NONE',  ( -2.500000000000000000, 0.000000000000000000, -2.300000000000000266 ) ) ;
#4544=CARTESIAN_POINT ( 'NONE',  ( -1.265664690411614835E-16, 2.066987299999999639, -1.949999998907525622 ) ) ;
#4552=ORIENTED_EDGE ( 'NONE', *, *, #1709, .T. ) ;
#4561=CARTESIAN_POINT ( 'NONE',  ( -1.035533905932738197, -2.500000000000000000, -1.343000000021849383 ) ) ;
#4564=CARTESIAN_POINT ( 'NONE',  ( 2.066987300000000083, -0.8561741729129449530, 1.092474635061568626E-09 ) ) ;
#4581=CARTESIAN_POINT ( 'NONE',  ( 1.767766952966368654, 1.767766952966369098, 0.6000000000000000888 ) ) ;
#4583=FILL_AREA_STYLE ('',( #9279 ) ) ;
#4593=CARTESIAN_POINT ( 'NONE',  ( 2.500000000000000000, 3.061616997868383141E-16, -1.799999997815050490 ) ) ;
#4602=CARTESIAN_POINT ( 'NONE',  ( 0.000000000000000000, 0.000000000000000000, 2.500000000000000000 ) ) ;
#4605=CARTESIAN_POINT ( 'NONE',  ( -1.265664690411614835E-16, 2.066987299999999639, 0.4500000010924747329 ) ) ;
#4609=( BOUNDED_CURVE ( )  B_SPLINE_CURVE ( 2, ( #13664, #7399, #5094, #12241, #14951, #6217, #9945, #11052, #1575 ),
 .UNSPECIFIED., .F., .F. ) 
 B_SPLINE_CURVE_WITH_KNOTS ( ( 3, 2, 2, 2, 3 ),
 ( 0.3571428571428571508, 0.3750000000000000000, 0.3928571428571428492, 0.4107142857142856984, 0.4285714285714285476 ),
 .UNSPECIFIED. ) 
 CURVE ( )  GEOMETRIC_REPRESENTATION_ITEM ( )  RATIONAL_B_SPLINE_CURVE ( ( 1.000000000000000000, 0.9238795325112867385, 1.000000000000000000, 0.9238795325112867385, 1.000000000000000000, 0.9238795325112867385, 1.000000000000000000, 0.9238795325112867385, 1.000000000000000000 ) ) 
 REPRESENTATION_ITEM ( '' )  );
#4618=CARTESIAN_POINT ( 'NONE',  ( 4.592425496802573972E-16, -2.500000000000000000, -1.199999997815050179 ) ) ;
#4622=CARTESIAN_POINT ( 'NONE',  ( 2.999999999999999556, 1.732050807568877859, -5.500000000000000000 ) ) ;
#4627=VECTOR ( 'NONE', #2522, 1000.000000000000000 ) ;
#4630=VERTEX_POINT ( 'NONE', #6734 ) ;
#4631=CARTESIAN_POINT ( 'NONE',  ( -2.066987299999999639, 0.8561741729129452860, 2.000000001092474555 ) ) ;
#4632=EDGE_CURVE ( 'NONE', #4630, #12887, #12834, .T. ) ;
#4636=CARTESIAN_POINT ( 'NONE',  ( -2.500000000000000444, 1.035533905932737753, -1.543000000021849338 ) ) ;
#4639=CARTESIAN_POINT ( 'NONE',  ( 1.461580736456472573, 1.461580736456472795, -0.6499999989075253559 ) ) ;
#4651=EDGE_CURVE ( 'NONE', #7968, #9805, #6812, .T. ) ;
#4677=CARTESIAN_POINT ( 'NONE',  ( -0.8561741729129455081, 2.066987299999999639, -0.2999999989075253226 ) ) ;
#4680=EDGE_CURVE ( 'NONE', #10824, #3215, #900, .T. ) ;
#4683=CARTESIAN_POINT ( 'NONE',  ( -3.000000000000000000, 1.732050807568877415, -5.500000000000000000 ) ) ;
#4686=CARTESIAN_POINT ( 'NONE',  ( -1.265664690411614835E-16, 2.066987299999999639, 1.250000001092474777 ) ) ;
#4688=EDGE_CURVE ( 'NONE', #4232, #5611, #6965, .T. ) ;
#4701=CARTESIAN_POINT ( 'NONE',  ( -1.767766952966368432, -1.767766952966369320, -1.299999997815050490 ) ) ;
#4713=CARTESIAN_POINT ( 'NONE',  ( -2.500000000000000000, 0.000000000000000000, -2.199999997815050623 ) ) ;
#4718=CARTESIAN_POINT ( 'NONE',  ( 2.500000000000000000, 3.061616997868383141E-16, -0.2930000000218493938 ) ) ;
#4722=CARTESIAN_POINT ( 'NONE',  ( -2.066987299999999639, 0.000000000000000000, -1.949999998907525178 ) ) ;
#4725=DIRECTION ( 'NONE',  ( 0.000000000000000000, 0.000000000000000000, 1.000000000000000000 ) ) ;
#4741=CARTESIAN_POINT ( 'NONE',  ( -1.084202172485504434E-16, 3.464101615137754830, -5.500000000000000000 ) ) ;
#4751=CARTESIAN_POINT ( 'NONE',  ( -2.500000000000000444, 1.035533905932737753, -0.7500000000000004441 ) ) ;
#4756=CARTESIAN_POINT ( 'NONE',  ( 0.8561741729129451750, 2.066987299999999639, 1.200000001092474733 ) ) ;
#4758=DIRECTION ( 'NONE',  ( 0.000000000000000000, 0.000000000000000000, -1.000000000000000000 ) ) ;
#4764=CARTESIAN_POINT ( 'NONE',  ( -2.066987299999999195, -0.8561741729129467293, -0.09999999890752520049 ) ) ;
#4775=LINE ( 'NONE', #8524, #8579 ) ;
#4795=CARTESIAN_POINT ( 'NONE',  ( -1.767766952966368432, -1.767766952966369320, -2.899999997815050357 ) ) ;
#4800=CARTESIAN_POINT ( 'NONE',  ( 2.500000000000000000, 3.061616997868383141E-16, -1.093000000021849605 ) ) ;
#4802=CARTESIAN_POINT ( 'NONE',  ( -1.461580736456472795, 1.461580736456472795, 2.150000001092474911 ) ) ;
#4805=LINE ( 'NONE', #14502, #2142 ) ;
#4819=CYLINDRICAL_SURFACE ( 'NONE', #8446, 2.500000000000000000 ) ;
#4821=CARTESIAN_POINT ( 'NONE',  ( -1.530808498934191571E-16, 2.500000000000000000, -2.500000000000000000 ) ) ;
#4837=CARTESIAN_POINT ( 'NONE',  ( 3.796994071234844259E-16, -2.066987299999999639, 0.05000000109247476621 ) ) ;
#4845=ADVANCED_FACE ( 'NONE', ( #13388 ), #14426, .F. ) ;
#4847=CARTESIAN_POINT ( 'NONE',  ( -2.066987299999999639, 0.000000000000000000, -0.9499999989075252893 ) ) ;
#4862=CARTESIAN_POINT ( 'NONE',  ( -1.530808498934191571E-16, 2.500000000000000000, -2.399999997815050801 ) ) ;
#4872=DIRECTION ( 'NONE',  ( -1.000000000000000000, 0.000000000000000000, 0.000000000000000000 ) ) ;
#4875=CARTESIAN_POINT ( 'NONE',  ( 1.461580736456472573, 1.461580736456472795, 0.9500000010924747329 ) ) ;
#4879=CARTESIAN_POINT ( 'NONE',  ( -2.500000000000000444, 1.035533905932737753, -2.343000000021849605 ) ) ;
#4882=CARTESIAN_POINT ( 'NONE',  ( 2.066987300000000083, -0.8561741729129449530, -1.599999998907525534 ) ) ;
#4917=B_SPLINE_CURVE_WITH_KNOTS ( 'NONE', 1,
 ( #12435, #9828 ),
 .UNSPECIFIED., .F., .F.,
 ( 2, 2 ),
 ( 0.000000000000000000, 1.000000000000000000 ),
 .UNSPECIFIED. ) ;
#4918=CARTESIAN_POINT ( 'NONE',  ( 0.8561741729129463963, -2.066987299999999195, 0.9000000010924746885 ) ) ;
#4925=CARTESIAN_POINT ( 'NONE',  ( -1.265664690411614835E-16, 2.066987299999999639, 2.050000001092474822 ) ) ;
#4932=ORIENTED_EDGE ( 'NONE', *, *, #12404, .F. ) ;
#4933=AXIS2_PLACEMENT_3D ( 'NONE', #81, #12012, #12248 ) ;
#4935=FACE_OUTER_BOUND ( 'NONE', #14312, .T. ) ;
#4950=VERTEX_POINT ( 'NONE', #1822 ) ;
#4956=CARTESIAN_POINT ( 'NONE',  ( 0.8561741729129463963, -2.066987299999999195, -0.8999999989075251339 ) ) ;
#4960=CARTESIAN_POINT ( 'NONE',  ( 1.767766952966368654, 1.767766952966369098, 1.399999999999999911 ) ) ;
#4964=CARTESIAN_POINT ( 'NONE',  ( 2.066987299999999639, 0.8561741729129456191, -1.499999998907525445 ) ) ;
#4980=CARTESIAN_POINT ( 'NONE',  ( -1.035533905932737753, 2.500000000000000444, -2.450000000000000178 ) ) ;
#4995=CARTESIAN_POINT ( 'NONE',  ( -1.461580736456472795, 1.461580736456472795, 0.5500000010924748217 ) ) ;
#5001=CARTESIAN_POINT ( 'NONE',  ( -2.066987299999999195, -0.8561741729129467293, -2.499999998907525001 ) ) ;
#5002=FACE_OUTER_BOUND ( 'NONE', #11159, .T. ) ;
#5004=CARTESIAN_POINT ( 'NONE',  ( -0.8561741729129455081, 2.066987299999999639, 1.900000001092474911 ) ) ;
#5028=CARTESIAN_POINT ( 'NONE',  ( 2.066987299999999639, 0.8561741729129456191, -0.6999999989075255113 ) ) ;
#5033=CARTESIAN_POINT ( 'NONE',  ( -2.500000000000000000, 0.000000000000000000, -2.293000000021850227 ) ) ;
#5039=CARTESIAN_POINT ( 'NONE',  ( -2.066987299999999195, -0.8561741729129466183, -1.099999998907525089 ) ) ;
#5072=CARTESIAN_POINT ( 'NONE',  ( 1.035533905932737531, 2.500000000000000444, 2.250000000000000444 ) ) ;
#5085=CARTESIAN_POINT ( 'NONE',  ( -1.084202172485504434E-15, -3.464101615137755275, -2.500000000000000000 ) ) ;
#5094=CARTESIAN_POINT ( 'NONE',  ( 1.767766952966369320, -1.767766952966368654, 0.3999999999999997446 ) ) ;
#5095=CARTESIAN_POINT ( 'NONE',  ( 2.500000000000000444, -1.035533905932737309, -2.649999997815050357 ) ) ;
#5101=EDGE_LOOP ( 'NONE', ( #2144, #5592, #10151, #14399 ) ) ;
#5103=ORIENTED_EDGE ( 'NONE', *, *, #6150, .F. ) ;
#5105=EDGE_LOOP ( 'NONE', ( #879, #10287, #15216, #2305 ) ) ;
#5106=DIRECTION ( 'NONE',  ( 0.000000000000000000, 0.000000000000000000, -1.000000000000000000 ) ) ;
#5108=CARTESIAN_POINT ( 'NONE',  ( -1.265664690411614835E-16, 2.066987299999999639, -1.349999998907525534 ) ) ;
#5112=CARTESIAN_POINT ( 'NONE',  ( -2.500000000000000000, -0.9567085809127248153, 2.546193976625564126 ) ) ;
#5116=CARTESIAN_POINT ( 'NONE',  ( -2.066987299999999639, 0.000000000000000000, 0.6500000010924747995 ) ) ;
#5149=CARTESIAN_POINT ( 'NONE',  ( -0.8561741729129455081, 2.066987299999999639, -2.699999998907525178 ) ) ;
#5154=CARTESIAN_POINT ( 'NONE',  ( -2.500000000000000000, 0.000000000000000000, -1.500000000000000000 ) ) ;
#5156=CARTESIAN_POINT ( 'NONE',  ( 2.066987299999999639, 2.531329380823229670E-16, -2.149999998907525356 ) ) ;
#5157=VECTOR ( 'NONE', #13478, 1000.000000000000000 ) ;
#5159=CARTESIAN_POINT ( 'NONE',  ( 1.461580736456473018, -1.461580736456472573, 1.550000001092474822 ) ) ;
#5174=CARTESIAN_POINT ( 'NONE',  ( -2.500000000000000444, 1.035533905932737753, -2.249999997815050001 ) ) ;
#5185=CARTESIAN_POINT ( 'NONE',  ( -0.8561741729129458411, -2.066987299999999195, 0.6000000010924746441 ) ) ;
#5190=CARTESIAN_POINT ( 'NONE',  ( -1.767766952966369098, 1.767766952966369098, -2.393000000021849427 ) ) ;
#5194=CARTESIAN_POINT ( 'NONE',  ( 1.461580736456473018, -1.461580736456472573, 0.9500000010924747329 ) ) ;
#5212=CARTESIAN_POINT ( 'NONE',  ( 2.500000000000000000, 3.061616997868383141E-16, 2.100000000000000089 ) ) ;
#5230=MANIFOLD_SOLID_BREP ( 'Thread1', #12830 ) ;
#5232=CARTESIAN_POINT ( 'NONE',  ( -1.035533905932737753, 2.500000000000000444, 2.350000000000000533 ) ) ;
#5240=CARTESIAN_POINT ( 'NONE',  ( 1.461580736456472573, 1.461580736456472795, -2.049999998907525267 ) ) ;
#5245=ADVANCED_FACE ( 'NONE', ( #4935 ), #14636, .T. ) ;
#5264=VERTEX_POINT ( 'NONE', #379 ) ;
#5269=CARTESIAN_POINT ( 'NONE',  ( -1.461580736456472351, -1.461580736456473018, 0.5500000010924748217 ) ) ;
#5273=CARTESIAN_POINT ( 'NONE',  ( -2.500000000000000444, 1.035533905932737753, 1.750000002184949999 ) ) ;
#5274=CARTESIAN_POINT ( 'NONE',  ( -2.500000000000000444, 1.035533905932737753, 2.449999999999999734 ) ) ;
#5277=CARTESIAN_POINT ( 'NONE',  ( 0.8561741729129463963, -2.066987299999999195, -1.499999998907525445 ) ) ;
#5280=AXIS2_PLACEMENT_3D ( 'NONE', #1479, #3789, #11113 ) ;
#5295=CARTESIAN_POINT ( 'NONE',  ( -1.035533905932737753, 2.500000000000000444, 2.356999999978150573 ) ) ;
#5305=SHAPE_REPRESENTATION ( 'pneumatic air inlet fitting', ( #14201 ), #6617 ) ;
#5314=CARTESIAN_POINT ( 'NONE',  ( -2.066987299999999195, -0.8561741729129466183, -1.699999998907525400 ) ) ;
#5328=EDGE_CURVE ( 'NONE', #13528, #7812, #12808, .T. ) ;
#5352=CARTESIAN_POINT ( 'NONE',  ( -1.035533905932737753, 2.500000000000000444, -0.8500000000000001998 ) ) ;
#5357=CARTESIAN_POINT ( 'NONE',  ( -2.500000000000000444, 1.035533905932737753, -0.6499999978150501345 ) ) ;
#5358=CARTESIAN_POINT ( 'NONE',  ( -0.8561741729129458411, -2.066987299999999195, -1.599999998907525534 ) ) ;
#5362=EDGE_LOOP ( 'NONE', ( #2793, #84, #11396, #7123 ) ) ;
#5370=CARTESIAN_POINT ( 'NONE',  ( -1.767766952966368432, -1.767766952966369320, -2.200000000000000178 ) ) ;
#5373=CARTESIAN_POINT ( 'NONE',  ( -2.500000000000000000, -0.4783542904563624076, 2.530096988290932547 ) ) ;
#5380=CARTESIAN_POINT ( 'NONE',  ( 2.236053883310440860, -1.154369717630873149, -2.500600154548837217 ) ) ;
#5390=CARTESIAN_POINT ( 'NONE',  ( 2.066987299999999639, 0.8561741729129456191, -1.299999998907525267 ) ) ;
#5397=CARTESIAN_POINT ( 'NONE',  ( -1.265664690411614835E-16, 2.066987299999999639, -0.5499999989075254891 ) ) ;
#5420=EDGE_LOOP ( 'NONE', ( #4468, #9881 ) ) ;
#5425=CARTESIAN_POINT ( 'NONE',  ( 2.066987299999999639, 2.531329380823229670E-16, -2.349999998907525534 ) ) ;
#5428=CARTESIAN_POINT ( 'NONE',  ( 1.767766952966368654, 1.767766952966369098, -0.2000000000000000944 ) ) ;
#5429=CARTESIAN_POINT ( 'NONE',  ( -2.500000000000000000, 0.000000000000000000, -0.7000000000000000666 ) ) ;
#5432=CARTESIAN_POINT ( 'NONE',  ( 2.066987300000000083, -0.8561741729129449530, 1.000000001092474777 ) ) ;
#5444=CARTESIAN_POINT ( 'NONE',  ( -2.500000000000000000, 0.000000000000000000, 1.800000002184949599 ) ) ;
#5446=CARTESIAN_POINT ( 'NONE',  ( 1.035533905932739085, -2.500000000000000000, -2.050000000000000266 ) ) ;
#5456=CARTESIAN_POINT ( 'NONE',  ( -0.5677240627250873528, 2.451883390204808055, -2.500792191741393555 ) ) ;
#5463=CYLINDRICAL_SURFACE ( 'NONE', #8884, 1.500000000000000000 ) ;
#5469=CARTESIAN_POINT ( 'NONE',  ( -2.500000000000000000, 0.000000000000000000, -0.7000000000000000666 ) ) ;
#5473=AXIS2_PLACEMENT_3D ( 'NONE', #5642, #3167, #14138 ) ;
#5477=CARTESIAN_POINT ( 'NONE',  ( -2.066987299999999195, -0.8561741729129467293, -0.2999999989075252671 ) ) ;
#5482=ORIENTED_EDGE ( 'NONE', *, *, #12795, .F. ) ;
#5505=CARTESIAN_POINT ( 'NONE',  ( 2.500000000000000000, 3.061616997868383141E-16, -1.900000000000000133 ) ) ;
#5518=CARTESIAN_POINT ( 'NONE',  ( 2.500000000000000444, 1.035533905932737975, 0.6500000021849496878 ) ) ;
#5519=EDGE_CURVE ( 'NONE', #6636, #8784, #2571, .T. ) ;
#5523=CARTESIAN_POINT ( 'NONE',  ( -1.530808498934191571E-16, 2.500000000000000000, 2.306999999978150306 ) ) ;
#5526=CARTESIAN_POINT ( 'NONE',  ( -1.461580736456472795, 1.461580736456472795, 0.3500000010924746996 ) ) ;
#5531=VERTEX_POINT ( 'NONE', #2356 ) ;
#5532=CARTESIAN_POINT ( 'NONE',  ( 2.483278259701947821, -0.3214162717929257562, -2.499187116769100658 ) ) ;
#5541=CARTESIAN_POINT ( 'NONE',  ( 1.767766984964215471, 1.767766920968521616, -2.500000000000000444 ) ) ;
#5543=CARTESIAN_POINT ( 'NONE',  ( -1.035533905932738197, -2.500000000000000000, -1.350000000000000089 ) ) ;
#5545=SURFACE_STYLE_USAGE ( .BOTH. , #15487 ) ;
#5553=CARTESIAN_POINT ( 'NONE',  ( 3.796994071234844259E-16, -2.066987299999999639, -1.749999998907525223 ) ) ;
#5584=CARTESIAN_POINT ( 'NONE',  ( 1.035533905932737531, 2.500000000000000444, -0.9500000000000001776 ) ) ;
#5588=CARTESIAN_POINT ( 'NONE',  ( -1.265664690411614835E-16, 2.066987299999999639, -2.749999998907525001 ) ) ;
#5591=MECHANICAL_DESIGN_GEOMETRIC_PRESENTATION_REPRESENTATION('',(#11677),#11178);
#5592=ORIENTED_EDGE ( 'NONE', *, *, #10914, .T. ) ;
#5595=FACE_BOUND ( 'NONE', #8329, .T. ) ;
#5598=CARTESIAN_POINT ( 'NONE',  ( -2.500000000000000000, 0.000000000000000000, 0.2000000021849495657 ) ) ;
#5602=CARTESIAN_POINT ( 'NONE',  ( -2.500000000000000444, 1.035533905932737753, 1.656999999978150617 ) ) ;
#5605=CARTESIAN_POINT ( 'NONE',  ( 1.461580736456473018, -1.461580736456472573, 0.7500000010924746663 ) ) ;
#5608=CARTESIAN_POINT ( 'NONE',  ( 1.767766952966368654, 1.767766952966369098, 0.7000000021849498433 ) ) ;
#5610=CARTESIAN_POINT ( 'NONE',  ( 1.035533905932739085, -2.500000000000000000, 0.4500000021849498433 ) ) ;
#5611=VERTEX_POINT ( 'NONE', #11105 ) ;
#5621=CARTESIAN_POINT ( 'NONE',  ( 2.500000000000000000, 3.061616997868383141E-16, -1.900000000000000133 ) ) ;
#5623=FACE_OUTER_BOUND ( 'NONE', #3601, .T. ) ;
#5629=ADVANCED_FACE ( 'NONE', ( #8335 ), #8505, .T. ) ;
#5630=CARTESIAN_POINT ( 'NONE',  ( 1.461580736456473018, -1.461580736456472573, -2.449999998907525622 ) ) ;
#5642=CARTESIAN_POINT ( 'NONE',  ( 0.000000000000000000, 0.000000000000000000, 2.500000000000000000 ) ) ;
#5645=CARTESIAN_POINT ( 'NONE',  ( -1.767766952966368432, -1.767766952966369320, 1.100000002184950088 ) ) ;
#5654=CARTESIAN_POINT ( 'NONE',  ( 2.500000000000000000, 3.061616997868383141E-16, 2.500000000000000000 ) ) ;
#5660=CARTESIAN_POINT ( 'NONE',  ( 1.767766952966368654, 1.767766952966369098, -0.8999999978150502455 ) ) ;
#5674=CARTESIAN_POINT ( 'NONE',  ( 2.500000000000000000, 3.061616997868383141E-16, -0.9999999978150503344 ) ) ;
#5679=CARTESIAN_POINT ( 'NONE',  ( 2.500000000000000444, 1.035533905932737975, -1.043000000021849560 ) ) ;
#5682=FACE_OUTER_BOUND ( 'NONE', #15685, .T. ) ;
#5687=CARTESIAN_POINT ( 'NONE',  ( -1.880234698852980557, -1.653780175538818620, -2.499419789153938698 ) ) ;
#5698=CARTESIAN_POINT ( 'NONE',  ( -2.500000000000000000, 0.000000000000000000, 1.700000000000000178 ) ) ;
#5699=CARTESIAN_POINT ( 'NONE',  ( 4.592425496802573972E-16, -2.500000000000000000, -1.300000000000000044 ) ) ;
#5701=CARTESIAN_POINT ( 'NONE',  ( -2.500000000000000000, 0.000000000000000000, 1.800000002184949821 ) ) ;
#5703=EDGE_CURVE ( 'NONE', #9607, #1897, #4420, .T. ) ;
#5716=FACE_OUTER_BOUND ( 'NONE', #3442, .T. ) ;
#5730=ORIENTED_EDGE ( 'NONE', *, *, #6320, .F. ) ;
#5736=CARTESIAN_POINT ( 'NONE',  ( -1.035533905932737753, 2.500000000000000444, 0.05000000218494983495 ) ) ;
#5747=ORIENTED_EDGE ( 'NONE', *, *, #8942, .T. ) ;
#5751=CARTESIAN_POINT ( 'NONE',  ( 1.035533905932737531, 2.500000000000000444, -0.8499999978150503122 ) ) ;
#5755=CARTESIAN_POINT ( 'NONE',  ( 2.500000000000000444, -1.035533905932737309, 0.4569999999781503286 ) ) ;
#5758=CARTESIAN_POINT ( 'NONE',  ( -1.461580736456472351, -1.461580736456473018, 1.350000001092474644 ) ) ;
#5765=VERTEX_POINT ( 'NONE', #6893 ) ;
#5776=CARTESIAN_POINT ( 'NONE',  ( -2.500000000000000444, 1.035533905932737753, 0.8500000000000001998 ) ) ;
#5777=CARTESIAN_POINT ( 'NONE',  ( -3.000000000000000444, -1.732050807568878081, -5.500000000000000000 ) ) ;
#5799=CARTESIAN_POINT ( 'NONE',  ( -1.461580736456472795, 1.461580736456472795, -0.2499999989075251672 ) ) ;
#5807=( BOUNDED_SURFACE ( )  B_SPLINE_SURFACE ( 1, 2, ( 
 ( #1848, #5373, #14094, #8061, #10217, #5295, #5523, #4323, #15070, #2896, #10370, #15221, #14021, #3128, #12821, #1925, #12592, #6798, #735, #5602, #4085, #10448, #15302, #4405, #3203, #1616, #6492, #8956, #13788, #8142, #8299, #3515, #9654, #8221, #14410, #6953, #11944, #14321, #10834, #12902, #15616, #10600, #13056, #5755, #2080, #14245, #9409, #4477, #15380, #15696, #2236, #7107, #1126, #2155, #2316, #6878, #5991, #13223, #4718, #9568, #7029, #887, #11785, #2003, #3278, #3354, #5834, #15460, #11857, #13137, #969, #1049, #9330, #5679, #4800, #5912, #15539, #11711, #10759, #4561, #8385, #10679, #3430, #4636, #9490, #7188, #812, #12027, #14495, #3593, #10526, #14173, #12977, #14575, #6235, #9811, #11150, #3902, #5033, #4879, #5190, #6313, #11071, #252, #9737 ),
 ( #5112, #3671, #12184, #1436, #13373, #2483, #12261, #7419, #10043, #1282, #17, #8548, #171, #1202, #9965, #6075, #14816, #9888, #8776, #7493, #14740, #1361, #3827, #7265, #4960, #11227, #14893, #13533, #6393, #13607, #7342, #6156, #10995, #14660, #13301, #8466, #2397, #8700, #94, #2719, #3748, #8624, #2641, #12340, #12102, #13459, #2562, #7571, #12419, #10919, #1517, #329, #1828, #560, #6702, #3032, #5428, #12653, #11457, #2798, #483, #6778, #713, #9091, #1904, #15204, #8934, #4064, #11306, #5352, #8856, #5584, #13689, #10273, #1672, #9165, #10198, #12802, #7962, #3108, #15125, #11613, #12573, #2876, #3979, #7648, #11532, #632, #4303, #12496, #5505, #10431, #4222, #9014, #7723, #6473, #6547, #13767, #11381, #15048, #13920, #6625, #14000, #4141, #1595 ),
 ( #7885, #13843, #403, #5273, #2955, #10349, #10121, #7803, #1751, #14973, #12726, #5974, #2299, #14228, #5816, #870, #4385, #9471, #11694, #1110, #4458, #2060, #12960, #12878, #6936, #14302, #9553, #14153, #2217, #9239, #14074, #8122, #7169, #14391, #3495, #8203, #11839, #5736, #13206, #1985, #3335, #9313, #12007, #15282, #3256, #3184, #10659, #7088, #11767, #794, #7009, #949, #3411, #15519, #10580, #11924, #5660, #15440, #8282, #8042, #6858, #10507, #4618, #4540, #4701, #9390, #8366, #15362, #13039, #13116, #2136, #1029, #5893, #10740, #15600, #2621, #8683, #6291, #3575, #7477, #2699, #11053, #75, #9719, #13282, #13358, #4862, #14556, #3652, #2546, #13443, #5095, #12167, #9946, #2463, #8529, #9793, #12243, #1343, #1264, #8447, #11132, #7326, #12321, #14798 ) ),
 .UNSPECIFIED., .F., .F., .F. ) 
 B_SPLINE_SURFACE_WITH_KNOTS ( ( 2, 1, 2 ),
 ( 3, 2, 2, 2, 2, 2, 2, 2, 2, 2, 2, 2, 2, 2, 2, 2, 2, 2, 2, 2, 2, 2, 2, 2, 2, 2, 2, 2, 2, 2, 2, 2, 2, 2, 2, 2, 2, 2, 2, 2, 2, 2, 2, 2, 2, 2, 2, 2, 2, 2, 2, 2, 3 ),
 ( -0.01000000000000000021, 0.000000000000000000, 1.000000000000000000 ),
 ( -0.008928571428571429811, 0.000000000000000000, 0.01785714285714285615, 0.03571428571428571230, 0.05357142857142856845, 0.07142857142857142461, 0.08928571428571428770, 0.1071428571428571369, 0.1250000000000000000, 0.1428571428571428492, 0.1607142857142857262, 0.1785714285714285754, 0.1964285714285714246, 0.2142857142857142738, 0.2321428571428571508, 0.2500000000000000000, 0.2678571428571428492, 0.2857142857142856984, 0.3035714285714285476, 0.3214285714285714524, 0.3392857142857143016, 0.3571428571428571508, 0.3750000000000000000, 0.3928571428571428492, 0.4107142857142856984, 0.4285714285714285476, 0.4464285714285714524, 0.4642857142857143016, 0.4821428571428571508, 0.5000000000000000000, 0.5178571428571429047, 0.5357142857142856984, 0.5535714285714286031, 0.5714285714285713969, 0.5892857142857143016, 0.6071428571428570953, 0.6250000000000000000, 0.6428571428571429047, 0.6607142857142856984, 0.6785714285714286031, 0.6964285714285713969, 0.7142857142857143016, 0.7321428571428570953, 0.7500000000000000000, 0.7678571428571429047, 0.7857142857142856984, 0.8035714285714286031, 0.8214285714285713969, 0.8392857142857143016, 0.8571428571428570953, 0.8750000000000000000, 0.8928571428571429047, 0.9018750000000000933 ),
 .UNSPECIFIED. ) 
 GEOMETRIC_REPRESENTATION_ITEM ( )  RATIONAL_B_SPLINE_SURFACE ( (
 ( 1.000000000000000000, 1.000000000000000000, 1.000000000000000000, 0.9238795325112867385, 1.000000000000000000, 0.9238795325112867385, 1.000000000000000000, 0.9238795325112867385, 1.000000000000000000, 0.9238795325112867385, 1.000000000000000000, 0.9238795325112867385, 1.000000000000000000, 0.9238795325112867385, 1.000000000000000000, 0.9238795325112867385, 1.000000000000000000, 0.9238795325112867385, 1.000000000000000000, 0.9238795325112867385, 1.000000000000000000, 0.9238795325112867385, 1.000000000000000000, 0.9238795325112867385, 1.000000000000000000, 0.9238795325112867385, 1.000000000000000000, 0.9238795325112867385, 1.000000000000000000, 0.9238795325112867385, 1.000000000000000000, 0.9238795325112867385, 1.000000000000000000, 0.9238795325112867385, 1.000000000000000000, 0.9238795325112867385, 1.000000000000000000, 0.9238795325112867385, 1.000000000000000000, 0.9238795325112867385, 1.000000000000000000, 0.9238795325112867385, 1.000000000000000000, 0.9238795325112867385, 1.000000000000000000, 0.9238795325112867385, 1.000000000000000000, 0.9238795325112867385, 1.000000000000000000, 0.9238795325112867385, 1.000000000000000000, 0.9238795325112867385, 1.000000000000000000, 0.9238795325112867385, 1.000000000000000000, 0.9238795325112867385, 1.000000000000000000, 0.9238795325112867385, 1.000000000000000000, 0.9238795325112867385, 1.000000000000000000, 0.9238795325112867385, 1.000000000000000000, 0.9238795325112867385, 1.000000000000000000, 0.9238795325112867385, 1.000000000000000000, 0.9238795325112867385, 1.000000000000000000, 0.9238795325112867385, 1.000000000000000000, 0.9238795325112867385, 1.000000000000000000, 0.9238795325112867385, 1.000000000000000000, 0.9238795325112867385, 1.000000000000000000, 0.9238795325112867385, 1.000000000000000000, 0.9238795325112867385, 1.000000000000000000, 0.9238795325112867385, 1.000000000000000000, 0.9238795325112867385, 1.000000000000000000, 0.9238795325112867385, 1.000000000000000000, 0.9238795325112867385, 1.000000000000000000, 0.9238795325112867385, 1.000000000000000000, 0.9238795325112867385, 1.000000000000000000, 0.9238795325112867385, 1.000000000000000000, 0.9238795325112867385, 1.000000000000000000, 0.9238795325112867385, 1.000000000000000000, 0.9238795325112867385, 1.000000000000000000, 0.9238795325112867385, 1.000000000000000000, 1.000000000000000000, 1.000000000000000000),
 ( 1.000000000000000000, 1.000000000000000000, 1.000000000000000000, 0.9238795325112867385, 1.000000000000000000, 0.9238795325112867385, 1.000000000000000000, 0.9238795325112867385, 1.000000000000000000, 0.9238795325112867385, 1.000000000000000000, 0.9238795325112867385, 1.000000000000000000, 0.9238795325112867385, 1.000000000000000000, 0.9238795325112867385, 1.000000000000000000, 0.9238795325112867385, 1.000000000000000000, 0.9238795325112867385, 1.000000000000000000, 0.9238795325112867385, 1.000000000000000000, 0.9238795325112867385, 1.000000000000000000, 0.9238795325112867385, 1.000000000000000000, 0.9238795325112867385, 1.000000000000000000, 0.9238795325112867385, 1.000000000000000000, 0.9238795325112867385, 1.000000000000000000, 0.9238795325112867385, 1.000000000000000000, 0.9238795325112867385, 1.000000000000000000, 0.9238795325112867385, 1.000000000000000000, 0.9238795325112867385, 1.000000000000000000, 0.9238795325112867385, 1.000000000000000000, 0.9238795325112867385, 1.000000000000000000, 0.9238795325112867385, 1.000000000000000000, 0.9238795325112867385, 1.000000000000000000, 0.9238795325112867385, 1.000000000000000000, 0.9238795325112867385, 1.000000000000000000, 0.9238795325112867385, 1.000000000000000000, 0.9238795325112867385, 1.000000000000000000, 0.9238795325112867385, 1.000000000000000000, 0.9238795325112867385, 1.000000000000000000, 0.9238795325112867385, 1.000000000000000000, 0.9238795325112867385, 1.000000000000000000, 0.9238795325112867385, 1.000000000000000000, 0.9238795325112867385, 1.000000000000000000, 0.9238795325112867385, 1.000000000000000000, 0.9238795325112867385, 1.000000000000000000, 0.9238795325112867385, 1.000000000000000000, 0.9238795325112867385, 1.000000000000000000, 0.9238795325112867385, 1.000000000000000000, 0.9238795325112867385, 1.000000000000000000, 0.9238795325112867385, 1.000000000000000000, 0.9238795325112867385, 1.000000000000000000, 0.9238795325112867385, 1.000000000000000000, 0.9238795325112867385, 1.000000000000000000, 0.9238795325112867385, 1.000000000000000000, 0.9238795325112867385, 1.000000000000000000, 0.9238795325112867385, 1.000000000000000000, 0.9238795325112867385, 1.000000000000000000, 0.9238795325112867385, 1.000000000000000000, 0.9238795325112867385, 1.000000000000000000, 0.9238795325112867385, 1.000000000000000000, 1.000000000000000000, 1.000000000000000000),
 ( 1.000000000000000000, 1.000000000000000000, 1.000000000000000000, 0.9238795325112867385, 1.000000000000000000, 0.9238795325112867385, 1.000000000000000000, 0.9238795325112867385, 1.000000000000000000, 0.9238795325112867385, 1.000000000000000000, 0.9238795325112867385, 1.000000000000000000, 0.9238795325112867385, 1.000000000000000000, 0.9238795325112867385, 1.000000000000000000, 0.9238795325112867385, 1.000000000000000000, 0.9238795325112867385, 1.000000000000000000, 0.9238795325112867385, 1.000000000000000000, 0.9238795325112867385, 1.000000000000000000, 0.9238795325112867385, 1.000000000000000000, 0.9238795325112867385, 1.000000000000000000, 0.9238795325112867385, 1.000000000000000000, 0.9238795325112867385, 1.000000000000000000, 0.9238795325112867385, 1.000000000000000000, 0.9238795325112867385, 1.000000000000000000, 0.9238795325112867385, 1.000000000000000000, 0.9238795325112867385, 1.000000000000000000, 0.9238795325112867385, 1.000000000000000000, 0.9238795325112867385, 1.000000000000000000, 0.9238795325112867385, 1.000000000000000000, 0.9238795325112867385, 1.000000000000000000, 0.9238795325112867385, 1.000000000000000000, 0.9238795325112867385, 1.000000000000000000, 0.9238795325112867385, 1.000000000000000000, 0.9238795325112867385, 1.000000000000000000, 0.9238795325112867385, 1.000000000000000000, 0.9238795325112867385, 1.000000000000000000, 0.9238795325112867385, 1.000000000000000000, 0.9238795325112867385, 1.000000000000000000, 0.9238795325112867385, 1.000000000000000000, 0.9238795325112867385, 1.000000000000000000, 0.9238795325112867385, 1.000000000000000000, 0.9238795325112867385, 1.000000000000000000, 0.9238795325112867385, 1.000000000000000000, 0.9238795325112867385, 1.000000000000000000, 0.9238795325112867385, 1.000000000000000000, 0.9238795325112867385, 1.000000000000000000, 0.9238795325112867385, 1.000000000000000000, 0.9238795325112867385, 1.000000000000000000, 0.9238795325112867385, 1.000000000000000000, 0.9238795325112867385, 1.000000000000000000, 0.9238795325112867385, 1.000000000000000000, 0.9238795325112867385, 1.000000000000000000, 0.9238795325112867385, 1.000000000000000000, 0.9238795325112867385, 1.000000000000000000, 0.9238795325112867385, 1.000000000000000000, 0.9238795325112867385, 1.000000000000000000, 0.9238795325112867385, 1.000000000000000000, 1.000000000000000000, 1.000000000000000000) ) ) 
 REPRESENTATION_ITEM ( '' )  SURFACE ( )  );
#5808=EDGE_CURVE ( 'NONE', #6636, #15622, #3216, .T. ) ;
#5816=CARTESIAN_POINT ( 'NONE',  ( 4.592425496802573972E-16, -2.500000000000000000, 1.200000002184949732 ) ) ;
#5820=CARTESIAN_POINT ( 'NONE',  ( 2.500000000000000000, 3.061616997868383141E-16, 0.5000000000000000000 ) ) ;
#5830=CARTESIAN_POINT ( 'NONE',  ( 1.767766952966369320, -1.767766952966368654, -1.899999997815050579 ) ) ;
#5834=CARTESIAN_POINT ( 'NONE',  ( -2.500000000000000000, 0.000000000000000000, -0.6930000000218496936 ) ) ;
#5837=CARTESIAN_POINT ( 'NONE',  ( 0.8561741729129451750, 2.066987299999999639, 0.2000000010924747329 ) ) ;
#5842=FACE_OUTER_BOUND ( 'NONE', #3582, .T. ) ;
#5849=ORIENTED_EDGE ( 'NONE', *, *, #771, .F. ) ;
#5851=UNCERTAINTY_MEASURE_WITH_UNIT (LENGTH_MEASURE( 1.000000000000000082E-05 ), #6210, 'distance_accuracy_value', 'NONE');
#5872=CARTESIAN_POINT ( 'NONE',  ( -1.461580736456472351, -1.461580736456473018, 1.550000001092474822 ) ) ;
#5880=CARTESIAN_POINT ( 'NONE',  ( 2.066987300000000083, -0.8561741729129450640, 1.000000001092474777 ) ) ;
#5882=ORIENTED_EDGE ( 'NONE', *, *, #5519, .F. ) ;
#5889=CARTESIAN_POINT ( 'NONE',  ( -2.500000000000000444, 1.035533905932737753, 0.1500000021849498544 ) ) ;
#5893=CARTESIAN_POINT ( 'NONE',  ( 1.767766952966368654, 1.767766952966369098, -1.699999997815050179 ) ) ;
#5900=VERTEX_POINT ( 'NONE', #14511 ) ;
#5908=CARTESIAN_POINT ( 'NONE',  ( -1.035533905932738197, -2.500000000000000000, -2.049999997815050268 ) ) ;
#5912=CARTESIAN_POINT ( 'NONE',  ( 2.500000000000000444, -1.035533905932737309, -1.143000000021849427 ) ) ;
#5915=CARTESIAN_POINT ( 'NONE',  ( 0.8561741729129463963, -2.066987299999999195, -0.8999999989075251339 ) ) ;
#5951=CARTESIAN_POINT ( 'NONE',  ( -2.066987299999999195, -0.8561741729129466183, -0.8999999989075251339 ) ) ;
#5959=CARTESIAN_POINT ( 'NONE',  ( 2.066987300000000083, -0.8561741729129450640, 0.2000000010924747329 ) ) ;
#5967=FILL_AREA_STYLE_COLOUR ( '', #7618 ) ;
#5974=CARTESIAN_POINT ( 'NONE',  ( 2.500000000000000444, -1.035533905932737309, 1.350000002184949643 ) ) ;
#5987=CARTESIAN_POINT ( 'NONE',  ( 4.592425496802573972E-16, -2.500000000000000000, -2.799999997815050268 ) ) ;
#5991=CARTESIAN_POINT ( 'NONE',  ( 1.767766952966368654, 1.767766952966369098, -0.1930000000218495826 ) ) ;
#5994=CARTESIAN_POINT ( 'NONE',  ( 2.066987299999999639, 2.531329380823229670E-16, 1.850000001092474866 ) ) ;
#5999=VERTEX_POINT ( 'NONE', #6409 ) ;
#6007=ADVANCED_FACE ( 'NONE', ( #12895 ), #8991, .T. ) ;
#6014=CARTESIAN_POINT ( 'NONE',  ( -2.500000000000000444, 1.035533905932737753, -2.350000000000000533 ) ) ;
#6017=PRODUCT ( 'pneumatic air inlet fitting', 'pneumatic air inlet fitting', '', ( #1850 ) ) ;
#6021=EDGE_CURVE ( 'NONE', #1290, #10824, #9011, .T. ) ;
#6032=CARTESIAN_POINT ( 'NONE',  ( 1.461580736456472573, 1.461580736456472795, 0.3500000010924749216 ) ) ;
#6040=CARTESIAN_POINT ( 'NONE',  ( 2.066987300000000083, -0.8561741729129450640, -0.5999999989075253115 ) ) ;
#6041=CARTESIAN_POINT ( 'NONE',  ( 0.000000000000000000, 0.000000000000000000, -5.500000000000000000 ) ) ;
#6046=CARTESIAN_POINT ( 'NONE',  ( -1.767766952966369098, 1.767766952966369098, 1.599999999999999867 ) ) ;
#6066=VERTEX_POINT ( 'NONE', #3470 ) ;
#6071=CARTESIAN_POINT ( 'NONE',  ( -2.066987299999999195, -0.8561741729129466183, 1.300000001092474600 ) ) ;
#6075=CARTESIAN_POINT ( 'NONE',  ( -1.035533905932738197, -2.500000000000000000, 1.849999999999999867 ) ) ;
#6077=CARTESIAN_POINT ( 'NONE',  ( -0.8561741729129455081, 2.066987299999999639, -1.299999998907525267 ) ) ;
#6082=VECTOR ( 'NONE', #2415, 1000.000000000000000 ) ;
#6086=ORIENTED_EDGE ( 'NONE', *, *, #6435, .T. ) ;
#6116=CARTESIAN_POINT ( 'NONE',  ( 0.8561741729129451750, 2.066987299999999639, -0.3999999989075250784 ) ) ;
#6126=CARTESIAN_POINT ( 'NONE',  ( -0.8561741729129455081, 2.066987299999999639, 0.5000000010924748883 ) ) ;
#6142=DIRECTION ( 'NONE',  ( -0.8660254037844385966, 0.5000000000000001110, 0.000000000000000000 ) ) ;
#6150=EDGE_CURVE ( 'NONE', #8455, #5900, #3783, .T. ) ;
#6152=CARTESIAN_POINT ( 'NONE',  ( -1.265664690411614835E-16, 2.066987299999999639, 1.850000001092474644 ) ) ;
#6154=CARTESIAN_POINT ( 'NONE',  ( 2.500000000000000444, 1.035533905932737975, -0.2500000000000002220 ) ) ;
#6156=CARTESIAN_POINT ( 'NONE',  ( -1.035533905932738197, -2.500000000000000000, 1.050000000000000044 ) ) ;
#6160=CARTESIAN_POINT ( 'NONE',  ( -1.461580736456472795, 1.461580736456472795, -2.049999998907525711 ) ) ;
#6194=CARTESIAN_POINT ( 'NONE',  ( -2.066987299999999639, 0.000000000000000000, 0.6500000010924747995 ) ) ;
#6196=VECTOR ( 'NONE', #1, 1000.000000000000000 ) ;
#6197=CARTESIAN_POINT ( 'NONE',  ( -3.000000000000000444, -1.732050807568878081, -5.500000000000000000 ) ) ;
#6203=ORIENTED_EDGE ( 'NONE', *, *, #4688, .T. ) ;
#6204=CARTESIAN_POINT ( 'NONE',  ( -1.461580736456472351, -1.461580736456473018, 1.350000001092474644 ) ) ;
#6210=( LENGTH_UNIT ( ) NAMED_UNIT ( * ) SI_UNIT ( .MILLI., .METRE. ) );
#6217=CARTESIAN_POINT ( 'NONE',  ( -1.035533905932738197, -2.500000000000000000, 0.2499999999999997780 ) ) ;
#6220=( BOUNDED_CURVE ( )  B_SPLINE_CURVE ( 2, ( #9929, #9778, #6438, #6274, #3942, #13736, #2681, #9851, #134 ),
 .UNSPECIFIED., .F., .F. ) 
 B_SPLINE_CURVE_WITH_KNOTS ( ( 3, 2, 2, 2, 3 ),
 ( 0.6428571428571429047, 0.6607142857142856984, 0.6785714285714286031, 0.6964285714285713969, 0.7142857142857143016 ),
 .UNSPECIFIED. ) 
 CURVE ( )  GEOMETRIC_REPRESENTATION_ITEM ( )  RATIONAL_B_SPLINE_CURVE ( ( 1.000000000000000000, 0.9238795325112867385, 1.000000000000000000, 0.9238795325112867385, 1.000000000000000000, 0.9238795325112867385, 1.000000000000000000, 0.9238795325112867385, 1.000000000000000000 ) ) 
 REPRESENTATION_ITEM ( '' )  );
#6231=CARTESIAN_POINT ( 'NONE',  ( 1.461580736456473018, -1.461580736456472573, -0.8499999989075254225 ) ) ;
#6233=LINE ( 'NONE', #10756, #9729 ) ;
#6235=CARTESIAN_POINT ( 'NONE',  ( 4.592425496802573972E-16, -2.500000000000000000, -2.093000000021849605 ) ) ;
#6239=CARTESIAN_POINT ( 'NONE',  ( 2.066987299999999639, 2.531329380823229670E-16, -1.549999998907525489 ) ) ;
#6245=( BOUNDED_CURVE ( )  B_SPLINE_CURVE ( 2, ( #14572, #9566, #8622, #8382, #9809, #3669, #14658, #6154, #8546 ),
 .UNSPECIFIED., .F., .F. ) 
 B_SPLINE_CURVE_WITH_KNOTS ( ( 3, 2, 2, 2, 3 ),
 ( 0.4285714285714285476, 0.4464285714285714524, 0.4642857142857143016, 0.4821428571428571508, 0.5000000000000000000 ),
 .UNSPECIFIED. ) 
 CURVE ( )  GEOMETRIC_REPRESENTATION_ITEM ( )  RATIONAL_B_SPLINE_CURVE ( ( 1.000000000000000000, 0.9238795325112867385, 1.000000000000000000, 0.9238795325112867385, 1.000000000000000000, 0.9238795325112867385, 1.000000000000000000, 0.9238795325112867385, 1.000000000000000000 ) ) 
 REPRESENTATION_ITEM ( '' )  );
#6262=ORIENTED_EDGE ( 'NONE', *, *, #6150, .T. ) ;
#6269=CARTESIAN_POINT ( 'NONE',  ( -2.066987299999999639, 0.000000000000000000, -1.749999998907525223 ) ) ;
#6272=DIRECTION ( 'NONE',  ( 0.000000000000000000, 0.000000000000000000, 1.000000000000000000 ) ) ;
#6274=CARTESIAN_POINT ( 'NONE',  ( 1.035533905932739085, -2.500000000000000000, -1.949999997815050401 ) ) ;
#6277=CARTESIAN_POINT ( 'NONE',  ( 2.500000000000000444, 1.035533905932737975, -2.549999997815050712 ) ) ;
#6279=CARTESIAN_POINT ( 'NONE',  ( -2.066987299999999639, 0.8561741729129455081, 0.4000000010924748550 ) ) ;
#6286=CARTESIAN_POINT ( 'NONE',  ( 2.500000000000000000, 3.061616997868383141E-16, -1.100000000000000311 ) ) ;
#6291=CARTESIAN_POINT ( 'NONE',  ( 1.035533905932739085, -2.500000000000000000, -1.949999997815050401 ) ) ;
#6308=CARTESIAN_POINT ( 'NONE',  ( 2.066987300000000083, -0.8561741729129449530, 1.092474635061568626E-09 ) ) ;
#6313=CARTESIAN_POINT ( 'NONE',  ( -1.035533905932737753, 2.500000000000000444, -2.443000000021850138 ) ) ;
#6317=CARTESIAN_POINT ( 'NONE',  ( 1.461580736456472573, 1.461580736456472795, 0.3500000010924749216 ) ) ;
#6320=EDGE_CURVE ( 'NONE', #6066, #3385, #2990, .T. ) ;
#6328=( BOUNDED_CURVE ( )  B_SPLINE_CURVE ( 2, ( #3499, #10821, #953, #9393, #12963, #14231, #13285, #9639, #5820 ),
 .UNSPECIFIED., .F., .F. ) 
 B_SPLINE_CURVE_WITH_KNOTS ( ( 3, 2, 2, 2, 3 ),
 ( 0.2857142857142856984, 0.3035714285714285476, 0.3214285714285714524, 0.3392857142857143016, 0.3571428571428571508 ),
 .UNSPECIFIED. ) 
 CURVE ( )  GEOMETRIC_REPRESENTATION_ITEM ( )  RATIONAL_B_SPLINE_CURVE ( ( 1.000000000000000000, 0.9238795325112867385, 1.000000000000000000, 0.9238795325112867385, 1.000000000000000000, 0.9238795325112867385, 1.000000000000000000, 0.9238795325112867385, 1.000000000000000000 ) ) 
 REPRESENTATION_ITEM ( '' )  );
#6342=ORIENTED_EDGE ( 'NONE', *, *, #10406, .T. ) ;
#6353=CARTESIAN_POINT ( 'NONE',  ( -1.530808498934191571E-16, 2.500000000000000000, 1.500000000000000000 ) ) ;
#6359=CARTESIAN_POINT ( 'NONE',  ( -1.461580736456472795, 1.461580736456472795, -1.849999998907525534 ) ) ;
#6362=CARTESIAN_POINT ( 'NONE',  ( 1.461580736456472573, 1.461580736456472795, 0.1500000010924747995 ) ) ;
#6377=LINE ( 'NONE', #13516, #14089 ) ;
#6382=ORIENTED_EDGE ( 'NONE', *, *, #7543, .T. ) ;
#6384=ORIENTED_EDGE ( 'NONE', *, *, #7368, .F. ) ;
#6389=CARTESIAN_POINT ( 'NONE',  ( -2.066987299999999639, 0.000000000000000000, 0.4500000010924747329 ) ) ;
#6393=CARTESIAN_POINT ( 'NONE',  ( 1.767766952966369320, -1.767766952966368654, 1.199999999999999956 ) ) ;
#6398=CARTESIAN_POINT ( 'NONE',  ( 2.066987299999999639, 0.8561741729129456191, -0.4999999989075253337 ) ) ;
#6409=CARTESIAN_POINT ( 'NONE',  ( 2.500000000000000000, 3.061616997868383141E-16, -0.9999999978150501123 ) ) ;
#6422=( BOUNDED_CURVE ( )  B_SPLINE_CURVE ( 2, ( #10417, #15267, #12865, #1969, #6847, #782, #5645, #3325, #15349 ),
 .UNSPECIFIED., .F., .F. ) 
 B_SPLINE_CURVE_WITH_KNOTS ( ( 3, 2, 2, 2, 3 ),
 ( 0.07142857142857142461, 0.08928571428571428770, 0.1071428571428571369, 0.1250000000000000000, 0.1428571428571428492 ),
 .UNSPECIFIED. ) 
 CURVE ( )  GEOMETRIC_REPRESENTATION_ITEM ( )  RATIONAL_B_SPLINE_CURVE ( ( 1.000000000000000000, 0.9238795325112867385, 1.000000000000000000, 0.9238795325112867385, 1.000000000000000000, 0.9238795325112867385, 1.000000000000000000, 0.9238795325112867385, 1.000000000000000000 ) ) 
 REPRESENTATION_ITEM ( '' )  );
#6429=VECTOR ( 'NONE', #631, 1000.000000000000114 ) ;
#6433=CARTESIAN_POINT ( 'NONE',  ( 4.592425496802573972E-16, -2.500000000000000000, 1.100000000000000089 ) ) ;
#6435=EDGE_CURVE ( 'NONE', #9302, #13528, #3169, .T. ) ;
#6438=CARTESIAN_POINT ( 'NONE',  ( 1.767766952966369320, -1.767766952966368654, -1.899999997815050357 ) ) ;
#6440=CARTESIAN_POINT ( 'NONE',  ( -2.066987299999999639, 0.8561741729129455081, -2.599999998907525089 ) ) ;
#6441=CARTESIAN_POINT ( 'NONE',  ( -1.767766952966369098, 1.767766952966369098, -3.099999997815050090 ) ) ;
#6469=CARTESIAN_POINT ( 'NONE',  ( 2.066987299999999639, 2.531329380823229670E-16, 0.05000000109247476621 ) ) ;
#6473=CARTESIAN_POINT ( 'NONE',  ( -1.035533905932738197, -2.500000000000000000, -2.150000000000000355 ) ) ;
#6476=CARTESIAN_POINT ( 'NONE',  ( 2.066987299999999639, 2.531329380823229670E-16, -1.349999998907525534 ) ) ;
#6484=EDGE_LOOP ( 'NONE', ( #5849, #14235, #10927, #12810 ) ) ;
#6492=CARTESIAN_POINT ( 'NONE',  ( 2.500000000000000000, 3.061616997868383141E-16, 1.306999999978150528 ) ) ;
#6509=CARTESIAN_POINT ( 'NONE',  ( -2.066987299999999195, -0.8561741729129466183, -2.499999998907525001 ) ) ;
#6516=CARTESIAN_POINT ( 'NONE',  ( -3.000000000000000444, -1.732050807568878081, -5.500000000000000000 ) ) ;
#6544=CARTESIAN_POINT ( 'NONE',  ( -2.066987299999999195, -0.8561741729129466183, -1.099999998907525089 ) ) ;
#6547=CARTESIAN_POINT ( 'NONE',  ( -1.767766952966368432, -1.767766952966369320, -2.200000000000000178 ) ) ;
#6548=CARTESIAN_POINT ( 'NONE',  ( -1.035533905932738197, -2.500000000000000000, -1.350000000000000089 ) ) ;
#6551=CARTESIAN_POINT ( 'NONE',  ( 1.461580736456472573, 1.461580736456472795, 1.150000001092474911 ) ) ;
#6557=FACE_OUTER_BOUND ( 'NONE', #7948, .T. ) ;
#6575=CARTESIAN_POINT ( 'NONE',  ( -1.767766952966368432, -1.767766952966369320, 0.3000000021849498211 ) ) ;
#6582=AXIS2_PLACEMENT_3D ( 'NONE', #10946, #11891, #3464 ) ;
#6584=CARTESIAN_POINT ( 'NONE',  ( 1.461580736456473018, -1.461580736456472573, -2.249999998907525445 ) ) ;
#6588=ADVANCED_FACE ( 'NONE', ( #7206 ), #4819, .T. ) ;
#6590=PRODUCT_DEFINITION_CONTEXT ( 'detailed design', #12674, 'design' ) ;
#6592=CARTESIAN_POINT ( 'NONE',  ( -1.035533905932738197, -2.500000000000000000, -2.849999997815050978 ) ) ;
#6593=CARTESIAN_POINT ( 'NONE',  ( -1.461580736456472795, 1.461580736456472795, -1.249999998907525223 ) ) ;
#6617=( GEOMETRIC_REPRESENTATION_CONTEXT ( 3 ) GLOBAL_UNCERTAINTY_ASSIGNED_CONTEXT ( ( #12617 ) ) GLOBAL_UNIT_ASSIGNED_CONTEXT ( ( #9056, #2915, #7766 ) ) REPRESENTATION_CONTEXT ( 'NONE', 'WORKASPACE' ) );
#6622=CARTESIAN_POINT ( 'NONE',  ( 1.461580736456473018, -1.461580736456472573, -2.449999998907525622 ) ) ;
#6625=CARTESIAN_POINT ( 'NONE',  ( -1.035533905932737753, 2.500000000000000444, -2.450000000000000178 ) ) ;
#6626=CARTESIAN_POINT ( 'NONE',  ( 2.500000000000000444, 1.035533905932737975, 2.149999999999999911 ) ) ;
#6630=CARTESIAN_POINT ( 'NONE',  ( -2.066987299999999195, -0.8561741729129466183, -1.699999998907525400 ) ) ;
#6636=VERTEX_POINT ( 'NONE', #14678 ) ;
#6641=CARTESIAN_POINT ( 'NONE',  ( 2.500000000000000444, 1.035533905932737975, 1.450000002184949732 ) ) ;
#6643=CARTESIAN_POINT ( 'NONE',  ( -1.035533905932738197, -2.500000000000000000, -2.150000000000000355 ) ) ;
#6652=AXIS2_PLACEMENT_3D ( 'NONE', #848, #14051, #3160 ) ;
#6662=CARTESIAN_POINT ( 'NONE',  ( -2.500000000000000000, -1.035533905932739307, 1.750000000000000000 ) ) ;
#6663=CARTESIAN_POINT ( 'NONE',  ( 1.767766952966369320, -1.767766952966368654, -0.4000000000000001887 ) ) ;
#6671=CARTESIAN_POINT ( 'NONE',  ( 0.8561741729129465073, -2.066987299999999195, -0.8999999989075251339 ) ) ;
#6680=CARTESIAN_POINT ( 'NONE',  ( 0.000000000000000000, 0.000000000000000000, 0.000000000000000000 ) ) ;
#6685=CARTESIAN_POINT ( 'NONE',  ( -1.461580736456472795, 1.461580736456472795, 2.150000001092474911 ) ) ;
#6698=CARTESIAN_POINT ( 'NONE',  ( -2.066987299999999639, 0.8561741729129452860, -2.799999998907525267 ) ) ;
#6702=CARTESIAN_POINT ( 'NONE',  ( -1.530808498934191571E-16, 2.500000000000000000, -0.1000000000000002554 ) ) ;
#6717=CARTESIAN_POINT ( 'NONE',  ( -1.767766952966368432, -1.767766952966369320, 1.100000002184949643 ) ) ;
#6719=CARTESIAN_POINT ( 'NONE',  ( -2.500000000000000000, 0.000000000000000000, -2.300000000000000266 ) ) ;
#6727=( BOUNDED_CURVE ( )  B_SPLINE_CURVE ( 2, ( #8098, #3231, #1003, #8013, #6833, #4275, #15497, #4355, #4593 ),
 .UNSPECIFIED., .F., .F. ) 
 B_SPLINE_CURVE_WITH_KNOTS ( ( 3, 2, 2, 2, 3 ),
 ( 0.5714285714285713969, 0.5892857142857143016, 0.6071428571428570953, 0.6250000000000000000, 0.6428571428571429047 ),
 .UNSPECIFIED. ) 
 CURVE ( )  GEOMETRIC_REPRESENTATION_ITEM ( )  RATIONAL_B_SPLINE_CURVE ( ( 1.000000000000000000, 0.9238795325112867385, 1.000000000000000000, 0.9238795325112867385, 1.000000000000000000, 0.9238795325112867385, 1.000000000000000000, 0.9238795325112867385, 1.000000000000000000 ) ) 
 REPRESENTATION_ITEM ( '' )  );
#6731=CARTESIAN_POINT ( 'NONE',  ( -2.340099644010926294, -0.9261024465269158679, -2.500002477042004401 ) ) ;
#6734=CARTESIAN_POINT ( 'NONE',  ( -2.500000000000000000, 0.000000000000000000, 0.2000000021849497878 ) ) ;
#6739=CARTESIAN_POINT ( 'NONE',  ( 1.767766952966369320, -1.767766952966368654, 2.000000000000000000 ) ) ;
#6740=CARTESIAN_POINT ( 'NONE',  ( -1.035533905932738197, -2.500000000000000000, 0.2499999999999997780 ) ) ;
#6749=CARTESIAN_POINT ( 'NONE',  ( 2.066987299999999639, 2.531329380823229670E-16, -2.349999998907525534 ) ) ;
#6778=CARTESIAN_POINT ( 'NONE',  ( 1.035533905932739085, -2.500000000000000000, -0.4499999999999998446 ) ) ;
#6783=CARTESIAN_POINT ( 'NONE',  ( -1.461580736456472351, -1.461580736456473018, -2.449999998907525178 ) ) ;
#6794=CARTESIAN_POINT ( 'NONE',  ( -1.035533905932738197, -2.500000000000000000, -0.4499999978150506230 ) ) ;
#6798=CARTESIAN_POINT ( 'NONE',  ( -2.500000000000000000, -1.035533905932739307, 1.756999999978150484 ) ) ;
#6802=CARTESIAN_POINT ( 'NONE',  ( -2.066987299999999639, 0.000000000000000000, 1.250000001092474777 ) ) ;
#6807=CARTESIAN_POINT ( 'NONE',  ( -2.067846033730325495, 1.412380013906880283, -2.500797151967781851 ) ) ;
#6808=CARTESIAN_POINT ( 'NONE',  ( -2.066987299999999195, -0.8561741729129467293, -0.8999999989075251339 ) ) ;
#6812=LINE ( 'NONE', #3291, #1259 ) ;
#6818=CARTESIAN_POINT ( 'NONE',  ( 1.035533905932737531, 2.500000000000000444, -1.750000000000000222 ) ) ;
#6819=CARTESIAN_POINT ( 'NONE',  ( 2.999999999999999556, 1.732050807568877859, -2.500000000000000000 ) ) ;
#6821=DIRECTION ( 'NONE',  ( -1.000000000000000000, 0.000000000000000000, 0.000000000000000000 ) ) ;
#6828=CARTESIAN_POINT ( 'NONE',  ( -2.066987299999999639, 0.8561741729129455081, -2.799999998907524823 ) ) ;
#6833=CARTESIAN_POINT ( 'NONE',  ( -1.530808498934191571E-16, 2.500000000000000000, -1.599999997815050312 ) ) ;
#6847=CARTESIAN_POINT ( 'NONE',  ( 4.592425496802573972E-16, -2.500000000000000000, 1.200000002184949732 ) ) ;
#6858=CARTESIAN_POINT ( 'NONE',  ( 1.767766952966369320, -1.767766952966368654, -1.099999997815050312 ) ) ;
#6861=CARTESIAN_POINT ( 'NONE',  ( 2.500000000000000000, 3.061616997868383141E-16, 1.300000000000000044 ) ) ;
#6867=ORIENTED_EDGE ( 'NONE', *, *, #9346, .F. ) ;
#6873=CARTESIAN_POINT ( 'NONE',  ( 1.767766952966368654, 1.767766952966369098, -0.8999999978150504676 ) ) ;
#6878=CARTESIAN_POINT ( 'NONE',  ( 1.035533905932737531, 2.500000000000000444, -0.1430000000218494827 ) ) ;
#6881=CARTESIAN_POINT ( 'NONE',  ( 2.066987300000000083, -0.8561741729129449530, 1.600000001092474644 ) ) ;
#6884=CARTESIAN_POINT ( 'NONE',  ( 2.500000000000000000, 3.061616997868383141E-16, 0.6000000021849497545 ) ) ;
#6893=CARTESIAN_POINT ( 'NONE',  ( -3.000000000000000000, 1.732050807568877415, -2.500000000000000000 ) ) ;
#6896=CARTESIAN_POINT ( 'NONE',  ( -1.767766952966369098, 1.767766952966369098, -1.600000000000000311 ) ) ;
#6901=CARTESIAN_POINT ( 'NONE',  ( 0.000000000000000000, 0.000000000000000000, 2.500000000000000000 ) ) ;
#6906=CARTESIAN_POINT ( 'NONE',  ( -1.265664690411614835E-16, 2.066987299999999639, -2.949999998907525178 ) ) ;
#6920=EDGE_CURVE ( 'NONE', #5611, #13777, #3031, .T. ) ;
#6921=CARTESIAN_POINT ( 'NONE',  ( 2.500000000000000000, 3.061616997868383141E-16, -1.900000000000000133 ) ) ;
#6936=CARTESIAN_POINT ( 'NONE',  ( 1.767766952966368654, 1.767766952966369098, 0.7000000021849498433 ) ) ;
#6948=ORIENTED_EDGE ( 'NONE', *, *, #7108, .F. ) ;
#6949=CARTESIAN_POINT ( 'NONE',  ( -1.035533905932738197, -2.500000000000000000, 1.150000002184949466 ) ) ;
#6953=CARTESIAN_POINT ( 'NONE',  ( -2.500000000000000444, 1.035533905932737753, 0.8569999999781505728 ) ) ;
#6959=CYLINDRICAL_SURFACE ( 'NONE', #7242, 2.500000000000000000 ) ;
#6960=ORIENTED_EDGE ( 'NONE', *, *, #11823, .F. ) ;
#6962=CIRCLE ( 'NONE', #93, 1.500000000000000222 ) ;
#6965=LINE ( 'NONE', #15314, #9626 ) ;
#6970=CARTESIAN_POINT ( 'NONE',  ( 1.767766952966369320, -1.767766952966368654, -1.099999997815050312 ) ) ;
#6971=CARTESIAN_POINT ( 'NONE',  ( -1.767766952966368432, -1.767766952966369320, 0.2000000000000000944 ) ) ;
#6996=FACE_OUTER_BOUND ( 'NONE', #1698, .T. ) ;
#6997=LINE ( 'NONE', #10494, #12861 ) ;
#7008=ADVANCED_FACE ( 'NONE', ( #948 ), #3574, .F. ) ;
#7009=CARTESIAN_POINT ( 'NONE',  ( -2.500000000000000000, 0.000000000000000000, -0.5999999978150503122 ) ) ;
#7020=DIRECTION ( 'NONE',  ( -0.8660254037844385966, 0.5000000000000001110, 0.000000000000000000 ) ) ;
#7025=CARTESIAN_POINT ( 'NONE',  ( -2.500000000000000000, 0.000000000000000000, -1.399999997815050579 ) ) ;
#7027=LINE ( 'NONE', #8059, #7216 ) ;
#7029=CARTESIAN_POINT ( 'NONE',  ( 1.767766952966369320, -1.767766952966368654, -0.3930000000218496492 ) ) ;
#7031=CARTESIAN_POINT ( 'NONE',  ( -1.461580736456472795, 1.461580736456472795, -0.4499999989075252338 ) ) ;
#7073=CARTESIAN_POINT ( 'NONE',  ( -0.8561741729129458411, -2.066987299999999195, 0.8000000010924748217 ) ) ;
#7075=ORIENTED_EDGE ( 'NONE', *, *, #11333, .F. ) ;
#7079=ORIENTED_EDGE ( 'NONE', *, *, #9722, .T. ) ;
#7088=CARTESIAN_POINT ( 'NONE',  ( -1.035533905932738197, -2.500000000000000000, -0.4499999978150504010 ) ) ;
#7089=DIRECTION ( 'NONE',  ( 0.000000000000000000, 0.000000000000000000, -1.000000000000000000 ) ) ;
#7101=CARTESIAN_POINT ( 'NONE',  ( -2.500000000000000000, -1.035533905932739307, -1.349999997815050312 ) ) ;
#7107=CARTESIAN_POINT ( 'NONE',  ( -2.500000000000000444, 1.035533905932737753, 0.05699999997815063946 ) ) ;
#7108=EDGE_CURVE ( 'NONE', #10844, #12887, #4609, .T. ) ;
#7123=ORIENTED_EDGE ( 'NONE', *, *, #12404, .T. ) ;
#7128=CARTESIAN_POINT ( 'NONE',  ( 4.592425496802573972E-16, -2.500000000000000000, -1.199999997815050179 ) ) ;
#7131=( NAMED_UNIT ( * ) SI_UNIT ( $, .STERADIAN. ) SOLID_ANGLE_UNIT ( ) );
#7147=CARTESIAN_POINT ( 'NONE',  ( 2.066987299999999639, 0.8561741729129456191, 1.900000001092474688 ) ) ;
#7154=CARTESIAN_POINT ( 'NONE',  ( 1.461580736456473018, -1.461580736456472573, 0.1500000010924746052 ) ) ;
#7169=CARTESIAN_POINT ( 'NONE',  ( -1.767766952966368432, -1.767766952966369320, 0.3000000021849498211 ) ) ;
#7184=CARTESIAN_POINT ( 'NONE',  ( -2.066987299999999639, 0.8561741729129452860, 1.200000001092474733 ) ) ;
#7186=DIRECTION ( 'NONE',  ( -0.8660254037844387076, -0.4999999999999998890, 0.000000000000000000 ) ) ;
#7188=CARTESIAN_POINT ( 'NONE',  ( -1.035533905932737753, 2.500000000000000444, -1.643000000021849205 ) ) ;
#7190=CARTESIAN_POINT ( 'NONE',  ( 1.461580736456473018, -1.461580736456472573, 1.750000001092474999 ) ) ;
#7206=FACE_OUTER_BOUND ( 'NONE', #14183, .T. ) ;
#7207=CARTESIAN_POINT ( 'NONE',  ( -1.035533905932738197, -2.500000000000000000, -1.249999997815050223 ) ) ;
#7211=EDGE_CURVE ( 'NONE', #338, #202, #9466, .T. ) ;
#7216=VECTOR ( 'NONE', #14243, 1000.000000000000000 ) ;
#7220=CYLINDRICAL_SURFACE ( 'NONE', #6582, 2.500000000000000000 ) ;
#7227=CARTESIAN_POINT ( 'NONE',  ( -1.265664690411614835E-16, 2.066987299999999639, 1.250000001092474777 ) ) ;
#7231=CARTESIAN_POINT ( 'NONE',  ( 2.500000000000000000, 3.061616997868383141E-16, -0.2999999999999999334 ) ) ;
#7234=CARTESIAN_POINT ( 'NONE',  ( 1.461580736456472573, 1.461580736456472795, 1.950000001092474955 ) ) ;
#7235=DIRECTION ( 'NONE',  ( 0.8660254037844385966, 0.4999999999999999445, 0.000000000000000000 ) ) ;
#7240=ORIENTED_EDGE ( 'NONE', *, *, #1713, .T. ) ;
#7242=AXIS2_PLACEMENT_3D ( 'NONE', #8556, #14583, #12033 ) ;
#7249=CARTESIAN_POINT ( 'NONE',  ( -2.500000000000000000, 0.000000000000000000, 0.9000000000000000222 ) ) ;
#7251=CARTESIAN_POINT ( 'NONE',  ( 1.035533905932737531, 2.500000000000000444, -2.449999997815050623 ) ) ;
#7260=ORIENTED_EDGE ( 'NONE', *, *, #11333, .T. ) ;
#7261=CARTESIAN_POINT ( 'NONE',  ( 0.8561741729129463963, -2.066987299999999195, 1.500000001092474555 ) ) ;
#7262=PLANE ( 'NONE',  #7810 ) ;
#7265=CARTESIAN_POINT ( 'NONE',  ( 1.035533905932737531, 2.500000000000000444, 1.450000000000000400 ) ) ;
#7270=CARTESIAN_POINT ( 'NONE',  ( 1.461580736456472573, 1.461580736456472795, 1.950000001092474955 ) ) ;
#7274=ORIENTED_EDGE ( 'NONE', *, *, #7211, .F. ) ;
#7303=CARTESIAN_POINT ( 'NONE',  ( -2.066987299999999639, 0.8561741729129452860, -0.1999999989075250117 ) ) ;
#7311=CARTESIAN_POINT ( 'NONE',  ( 2.066987299999999639, 0.8561741729129456191, 0.3000000010924747662 ) ) ;
#7326=CARTESIAN_POINT ( 'NONE',  ( -1.530808498934191571E-16, 2.500000000000000000, -3.199999997815050623 ) ) ;
#7331=CARTESIAN_POINT ( 'NONE',  ( 1.767766984964215471, 1.767766920968521616, -2.500000000000000444 ) ) ;
#7338=CARTESIAN_POINT ( 'NONE',  ( 1.461580736456473018, -1.461580736456472573, 1.550000001092474822 ) ) ;
#7342=CARTESIAN_POINT ( 'NONE',  ( 4.592425496802573972E-16, -2.500000000000000000, 1.100000000000000089 ) ) ;
#7345=CARTESIAN_POINT ( 'NONE',  ( -1.461580736456472351, -1.461580736456473018, -1.849999998907525534 ) ) ;
#7368=EDGE_CURVE ( 'NONE', #4232, #2808, #6233, .T. ) ;
#7371=EDGE_CURVE ( 'NONE', #12887, #5264, #6245, .T. ) ;
#7374=CARTESIAN_POINT ( 'NONE',  ( -1.500000000000000222, 0.000000000000000000, -5.500000000000000000 ) ) ;
#7378=CARTESIAN_POINT ( 'NONE',  ( -1.461580736456472795, 1.461580736456472795, -1.049999998907525045 ) ) ;
#7385=CARTESIAN_POINT ( 'NONE',  ( 2.066987299999999639, 2.531329380823229670E-16, -0.5499999989075250451 ) ) ;
#7399=CARTESIAN_POINT ( 'NONE',  ( 2.500000000000000444, -1.035533905932737309, 0.4499999999999999556 ) ) ;
#7403=CARTESIAN_POINT ( 'NONE',  ( -1.530808498934191571E-16, 2.500000000000000000, -2.399999997815050801 ) ) ;
#7415=CARTESIAN_POINT ( 'NONE',  ( 1.461580736456472573, 1.461580736456472795, -0.6499999989075253559 ) ) ;
#7419=CARTESIAN_POINT ( 'NONE',  ( 1.035533905932737531, 2.500000000000000444, 2.250000000000000444 ) ) ;
#7422=CARTESIAN_POINT ( 'NONE',  ( -2.066987299999999195, -0.8561741729129466183, -2.699999998907525178 ) ) ;
#7431=( BOUNDED_CURVE ( )  B_SPLINE_CURVE ( 2, ( #1483, #11275, #11352, #5004, #7696, #374, #3948, #12621, #2924, #14784, #5159, #15021, #8985, #9933, #6204, #10013, #4029, #2766, #9857, #10166, #14708, #1642, #4113, #13813, #3871, #8744, #11041, #139, #7774, #3796, #2606, #7464, #12306, #6279, #11119, #8823, #222, #7538, #6362, #7620, #12464, #1566, #765, #13972, #9062, #4193, #15408, #5477, #8093, #3001, #3228, #12699, #5397, #10477, #12931, #12850, #10400, #3078, #14046, #6671, #1718, #8170, #4506, #679, #8010, #7926, #6593, #11663, #13889, #3309, #11504, #4271, #605, #1796, #10320, #15172, #5553, #528, #9137, #2031, #9286, #12770, #9361, #7857, #15251, #1874, #14200, #11428, #6749, #11582, #5630, #10246, #4352, #9210, #3155, #1953, #15332, #6828, #4429, #14122, #6906 ),
 .UNSPECIFIED., .F., .F. ) 
 B_SPLINE_CURVE_WITH_KNOTS ( ( 3, 2, 2, 2, 2, 2, 2, 2, 2, 2, 2, 2, 2, 2, 2, 2, 2, 2, 2, 2, 2, 2, 2, 2, 2, 2, 2, 2, 2, 2, 2, 2, 2, 2, 2, 2, 2, 2, 2, 2, 2, 2, 2, 2, 2, 2, 2, 2, 2, 2, 3 ),
 ( 0.000000000000000000, 0.01785714285714285615, 0.03571428571428571230, 0.05357142857142856845, 0.07142857142857142461, 0.08928571428571428770, 0.1071428571428571369, 0.1250000000000000000, 0.1428571428571428492, 0.1607142857142857262, 0.1785714285714285754, 0.1964285714285714246, 0.2142857142857142738, 0.2321428571428571508, 0.2500000000000000000, 0.2678571428571428492, 0.2857142857142856984, 0.3035714285714285476, 0.3214285714285714524, 0.3392857142857143016, 0.3571428571428571508, 0.3750000000000000000, 0.3928571428571428492, 0.4107142857142856984, 0.4285714285714285476, 0.4464285714285714524, 0.4642857142857143016, 0.4821428571428571508, 0.5000000000000000000, 0.5178571428571429047, 0.5357142857142856984, 0.5535714285714286031, 0.5714285714285713969, 0.5892857142857143016, 0.6071428571428570953, 0.6250000000000000000, 0.6428571428571429047, 0.6607142857142856984, 0.6785714285714286031, 0.6964285714285715079, 0.7142857142857143016, 0.7321428571428570953, 0.7500000000000000000, 0.7678571428571429047, 0.7857142857142856984, 0.8035714285714286031, 0.8214285714285713969, 0.8392857142857143016, 0.8571428571428570953, 0.8750000000000000000, 0.8928571428571429047 ),
 .UNSPECIFIED. ) 
 CURVE ( )  GEOMETRIC_REPRESENTATION_ITEM ( )  RATIONAL_B_SPLINE_CURVE ( ( 1.000000000000000000, 0.9238795325112867385, 1.000000000000000000, 0.9238795325112867385, 1.000000000000000000, 0.9238795325112867385, 1.000000000000000000, 0.9238795325112867385, 1.000000000000000000, 0.9238795325112867385, 1.000000000000000000, 0.9238795325112867385, 1.000000000000000000, 0.9238795325112867385, 1.000000000000000000, 0.9238795325112867385, 1.000000000000000000, 0.9238795325112867385, 1.000000000000000000, 0.9238795325112867385, 1.000000000000000000, 0.9238795325112867385, 1.000000000000000000, 0.9238795325112867385, 1.000000000000000000, 0.9238795325112867385, 1.000000000000000000, 0.9238795325112867385, 1.000000000000000000, 0.9238795325112867385, 1.000000000000000000, 0.9238795325112867385, 1.000000000000000000, 0.9238795325112867385, 1.000000000000000000, 0.9238795325112867385, 1.000000000000000000, 0.9238795325112867385, 1.000000000000000000, 0.9238795325112867385, 1.000000000000000000, 0.9238795325112867385, 1.000000000000000000, 0.9238795325112867385, 1.000000000000000000, 0.9238795325112867385, 1.000000000000000000, 0.9238795325112867385, 1.000000000000000000, 0.9238795325112867385, 1.000000000000000000, 0.9238795325112867385, 1.000000000000000000, 0.9238795325112867385, 1.000000000000000000, 0.9238795325112867385, 1.000000000000000000, 0.9238795325112867385, 1.000000000000000000, 0.9238795325112867385, 1.000000000000000000, 0.9238795325112867385, 1.000000000000000000, 0.9238795325112867385, 1.000000000000000000, 0.9238795325112867385, 1.000000000000000000, 0.9238795325112867385, 1.000000000000000000, 0.9238795325112867385, 1.000000000000000000, 0.9238795325112867385, 1.000000000000000000, 0.9238795325112867385, 1.000000000000000000, 0.9238795325112867385, 1.000000000000000000, 0.9238795325112867385, 1.000000000000000000, 0.9238795325112867385, 1.000000000000000000, 0.9238795325112867385, 1.000000000000000000, 0.9238795325112867385, 1.000000000000000000, 0.9238795325112867385, 1.000000000000000000, 0.9238795325112867385, 1.000000000000000000, 0.9238795325112867385, 1.000000000000000000, 0.9238795325112867385, 1.000000000000000000, 0.9238795325112867385, 1.000000000000000000, 0.9238795325112867385, 1.000000000000000000, 0.9238795325112867385, 1.000000000000000000, 0.9238795325112867385, 1.000000000000000000 ) ) 
 REPRESENTATION_ITEM ( '' )  );
#7437=CARTESIAN_POINT ( 'NONE',  ( -2.500000000000000000, 0.000000000000000000, 2.500000000000000000 ) ) ;
#7438=LINE ( 'NONE', #8648, #5157 ) ;
#7451=CARTESIAN_POINT ( 'NONE',  ( 0.8561741729129463963, -2.066987299999999195, -2.299999998907525267 ) ) ;
#7456=CARTESIAN_POINT ( 'NONE',  ( -2.500000000000000000, -1.035533905932739307, -0.6500000000000000222 ) ) ;
#7464=CARTESIAN_POINT ( 'NONE',  ( -2.066987299999999195, -0.8561741729129467293, 0.5000000010924746663 ) ) ;
#7477=CARTESIAN_POINT ( 'NONE',  ( -1.035533905932738197, -2.500000000000000000, -2.049999997815050268 ) ) ;
#7489=CARTESIAN_POINT ( 'NONE',  ( -1.461580736456472795, 1.461580736456472795, -0.4499999989075252338 ) ) ;
#7493=CARTESIAN_POINT ( 'NONE',  ( -2.500000000000000444, 1.035533905932737753, 1.649999999999999911 ) ) ;
#7498=CARTESIAN_POINT ( 'NONE',  ( -1.461580736456472351, -1.461580736456473018, 0.7500000010924748883 ) ) ;
#7528=CARTESIAN_POINT ( 'NONE',  ( 2.066987300000000083, -0.8561741729129449530, -2.199999998907525178 ) ) ;
#7535=CARTESIAN_POINT ( 'NONE',  ( 1.461580736456472573, 1.461580736456472795, -1.249999998907525223 ) ) ;
#7538=CARTESIAN_POINT ( 'NONE',  ( 0.8561741729129452860, 2.066987299999999639, 0.2000000010924747329 ) ) ;
#7543=EDGE_CURVE ( 'NONE', #1570, #4950, #13396, .T. ) ;
#7556=EDGE_LOOP ( 'NONE', ( #13215, #9748, #11604 ) ) ;
#7567=CARTESIAN_POINT ( 'NONE',  ( -2.066987299999999639, 0.8561741729129452860, -1.999999998907524779 ) ) ;
#7571=CARTESIAN_POINT ( 'NONE',  ( -1.035533905932738197, -2.500000000000000000, 0.2499999999999997780 ) ) ;
#7575=CARTESIAN_POINT ( 'NONE',  ( -1.461580736456472351, -1.461580736456473018, -0.8499999989075254225 ) ) ;
#7608=CARTESIAN_POINT ( 'NONE',  ( -2.066987299999999639, 0.8561741729129452860, -2.599999998907525089 ) ) ;
#7617=CARTESIAN_POINT ( 'NONE',  ( -0.8561741729129458411, -2.066987299999999195, -2.399999998907525356 ) ) ;
#7618=COLOUR_RGB ( '', 0.31764706, 0.68627451, 0.89019608) ;
#7620=CARTESIAN_POINT ( 'NONE',  ( 2.066987299999999639, 0.8561741729129456191, 0.1000000010924746996 ) ) ;
#7642=CARTESIAN_POINT ( 'NONE',  ( 0.000000000000000000, 0.000000000000000000, 2.500000000000000000 ) ) ;
#7644=CARTESIAN_POINT ( 'NONE',  ( -1.461580736456472795, 1.461580736456472795, -1.249999998907525223 ) ) ;
#7648=CARTESIAN_POINT ( 'NONE',  ( -1.035533905932737753, 2.500000000000000444, -1.649999999999999911 ) ) ;
#7652=CARTESIAN_POINT ( 'NONE',  ( 2.066987299999999639, 2.531329380823229670E-16, 1.050000001092474822 ) ) ;
#7658=ORIENTED_EDGE ( 'NONE', *, *, #6021, .T. ) ;
#7659=EDGE_LOOP ( 'NONE', ( #13274, #2390, #14418, #5730 ) ) ;
#7685=CARTESIAN_POINT ( 'NONE',  ( -1.767766952966368432, -1.767766952966369320, 1.800000000000000044 ) ) ;
#7686=LINE ( 'NONE', #6819, #59 ) ;
#7692=DIRECTION ( 'NONE',  ( 0.000000000000000000, 0.000000000000000000, -1.000000000000000000 ) ) ;
#7696=CARTESIAN_POINT ( 'NONE',  ( -1.265664690411614835E-16, 2.066987299999999639, 1.850000001092474644 ) ) ;
#7720=CARTESIAN_POINT ( 'NONE',  ( -2.066987299999999639, 0.000000000000000000, -1.149999998907525356 ) ) ;
#7723=CARTESIAN_POINT ( 'NONE',  ( 4.592425496802573972E-16, -2.500000000000000000, -2.100000000000000089 ) ) ;
#7728=CARTESIAN_POINT ( 'NONE',  ( -1.265664690411614835E-16, 2.066987299999999639, 0.4500000010924747329 ) ) ;
#7733=( BOUNDED_SURFACE ( )  B_SPLINE_SURFACE ( 1, 2, ( 
 ( #14097, #8146, #9185, #12906, #654, #8301, #3131, #10374, #10529, #6881, #890, #972, #15224, #11789, #5758, #12824, #6802, #4327, #9334, #3356, #815, #2158, #2007, #15462, #9493, #11714, #5605, #11637, #7984, #15304, #10452, #3205, #15383, #10603, #5526, #1928, #739, #5837, #12980, #4408, #9261, #4564, #9414, #4480, #13139, #14326, #14175, #8225, #3283, #14249, #7031, #11860, #10682, #15543, #4639, #3433, #2239, #175, #13463, #5915, #8388, #1365, #10763, #5039, #12265, #3753, #8628, #6077, #15700, #2565, #1206, #4964, #6239, #4882, #14498, #13303, #12187, #2402, #7345, #14413, #4722, #9892, #6160, #14578, #1052, #8703, #14745, #98, #9658, #10837, #1286, #9740, #11075, #15618, #1129, #7422, #3831, #3675, #9571, #13537, #2646 ),
 ( #12030, #11947, #4802, #8553, #3518, #21, #7270, #10998, #5994, #3595, #7190, #12105, #13226, #13377, #2318, #8471, #2487, #9816, #10921, #14664, #12579, #13924, #6551, #4147, #7652, #5432, #5194, #14978, #256, #3982, #7498, #15132, #5116, #1439, #1598, #13693, #7728, #7808, #6317, #8939, #2881, #3906, #13610, #11154, #407, #10203, #12500, #9020, #8861, #11386, #565, #2803, #12422, #2723, #9970, #6398, #1522, #10048, #14896, #13772, #12344, #14820, #7575, #12659, #4069, #8781, #11231, #1676, #487, #333, #4226, #10278, #6476, #15053, #11310, #5277, #10126, #5358, #13846, #6630, #2959, #1756, #11463, #9095, #4544, #12729, #15208, #8207, #1832, #11843, #3339, #10584, #15445, #12883, #6783, #9394, #8046, #11771, #13043, #11698, #5588 ) ),
 .UNSPECIFIED., .F., .F., .F. ) 
 B_SPLINE_SURFACE_WITH_KNOTS ( ( 2, 2 ),
 ( 3, 2, 2, 2, 2, 2, 2, 2, 2, 2, 2, 2, 2, 2, 2, 2, 2, 2, 2, 2, 2, 2, 2, 2, 2, 2, 2, 2, 2, 2, 2, 2, 2, 2, 2, 2, 2, 2, 2, 2, 2, 2, 2, 2, 2, 2, 2, 2, 2, 2, 3 ),
 ( 0.000000000000000000, 1.000000000000000000 ),
 ( 0.000000000000000000, 0.01785714285714285615, 0.03571428571428571230, 0.05357142857142856845, 0.07142857142857142461, 0.08928571428571428770, 0.1071428571428571369, 0.1250000000000000000, 0.1428571428571428492, 0.1607142857142857262, 0.1785714285714285754, 0.1964285714285714246, 0.2142857142857142738, 0.2321428571428571508, 0.2500000000000000000, 0.2678571428571428492, 0.2857142857142856984, 0.3035714285714285476, 0.3214285714285714524, 0.3392857142857143016, 0.3571428571428571508, 0.3750000000000000000, 0.3928571428571428492, 0.4107142857142856984, 0.4285714285714285476, 0.4464285714285714524, 0.4642857142857143016, 0.4821428571428571508, 0.5000000000000000000, 0.5178571428571429047, 0.5357142857142856984, 0.5535714285714286031, 0.5714285714285713969, 0.5892857142857143016, 0.6071428571428570953, 0.6250000000000000000, 0.6428571428571429047, 0.6607142857142856984, 0.6785714285714286031, 0.6964285714285713969, 0.7142857142857143016, 0.7321428571428570953, 0.7500000000000000000, 0.7678571428571429047, 0.7857142857142856984, 0.8035714285714286031, 0.8214285714285713969, 0.8392857142857143016, 0.8571428571428570953, 0.8750000000000000000, 0.8928571428571429047 ),
 .UNSPECIFIED. ) 
 GEOMETRIC_REPRESENTATION_ITEM ( )  RATIONAL_B_SPLINE_SURFACE ( (
 ( 1.000000000000000000, 0.9238795325112867385, 1.000000000000000000, 0.9238795325112867385, 1.000000000000000000, 0.9238795325112867385, 1.000000000000000000, 0.9238795325112867385, 1.000000000000000000, 0.9238795325112867385, 1.000000000000000000, 0.9238795325112867385, 1.000000000000000000, 0.9238795325112867385, 1.000000000000000000, 0.9238795325112867385, 1.000000000000000000, 0.9238795325112867385, 1.000000000000000000, 0.9238795325112867385, 1.000000000000000000, 0.9238795325112867385, 1.000000000000000000, 0.9238795325112867385, 1.000000000000000000, 0.9238795325112867385, 1.000000000000000000, 0.9238795325112867385, 1.000000000000000000, 0.9238795325112867385, 1.000000000000000000, 0.9238795325112867385, 1.000000000000000000, 0.9238795325112867385, 1.000000000000000000, 0.9238795325112867385, 1.000000000000000000, 0.9238795325112867385, 1.000000000000000000, 0.9238795325112867385, 1.000000000000000000, 0.9238795325112867385, 1.000000000000000000, 0.9238795325112867385, 1.000000000000000000, 0.9238795325112867385, 1.000000000000000000, 0.9238795325112867385, 1.000000000000000000, 0.9238795325112867385, 1.000000000000000000, 0.9238795325112867385, 1.000000000000000000, 0.9238795325112867385, 1.000000000000000000, 0.9238795325112867385, 1.000000000000000000, 0.9238795325112867385, 1.000000000000000000, 0.9238795325112867385, 1.000000000000000000, 0.9238795325112867385, 1.000000000000000000, 0.9238795325112867385, 1.000000000000000000, 0.9238795325112867385, 1.000000000000000000, 0.9238795325112867385, 1.000000000000000000, 0.9238795325112867385, 1.000000000000000000, 0.9238795325112867385, 1.000000000000000000, 0.9238795325112867385, 1.000000000000000000, 0.9238795325112867385, 1.000000000000000000, 0.9238795325112867385, 1.000000000000000000, 0.9238795325112867385, 1.000000000000000000, 0.9238795325112867385, 1.000000000000000000, 0.9238795325112867385, 1.000000000000000000, 0.9238795325112867385, 1.000000000000000000, 0.9238795325112867385, 1.000000000000000000, 0.9238795325112867385, 1.000000000000000000, 0.9238795325112867385, 1.000000000000000000, 0.9238795325112867385, 1.000000000000000000, 0.9238795325112867385, 1.000000000000000000, 0.9238795325112867385, 1.000000000000000000, 0.9238795325112867385, 1.000000000000000000),
 ( 1.000000000000000000, 0.9238795325112867385, 1.000000000000000000, 0.9238795325112867385, 1.000000000000000000, 0.9238795325112867385, 1.000000000000000000, 0.9238795325112867385, 1.000000000000000000, 0.9238795325112867385, 1.000000000000000000, 0.9238795325112867385, 1.000000000000000000, 0.9238795325112867385, 1.000000000000000000, 0.9238795325112867385, 1.000000000000000000, 0.9238795325112867385, 1.000000000000000000, 0.9238795325112867385, 1.000000000000000000, 0.9238795325112867385, 1.000000000000000000, 0.9238795325112867385, 1.000000000000000000, 0.9238795325112867385, 1.000000000000000000, 0.9238795325112867385, 1.000000000000000000, 0.9238795325112867385, 1.000000000000000000, 0.9238795325112867385, 1.000000000000000000, 0.9238795325112867385, 1.000000000000000000, 0.9238795325112867385, 1.000000000000000000, 0.9238795325112867385, 1.000000000000000000, 0.9238795325112867385, 1.000000000000000000, 0.9238795325112867385, 1.000000000000000000, 0.9238795325112867385, 1.000000000000000000, 0.9238795325112867385, 1.000000000000000000, 0.9238795325112867385, 1.000000000000000000, 0.9238795325112867385, 1.000000000000000000, 0.9238795325112867385, 1.000000000000000000, 0.9238795325112867385, 1.000000000000000000, 0.9238795325112867385, 1.000000000000000000, 0.9238795325112867385, 1.000000000000000000, 0.9238795325112867385, 1.000000000000000000, 0.9238795325112867385, 1.000000000000000000, 0.9238795325112867385, 1.000000000000000000, 0.9238795325112867385, 1.000000000000000000, 0.9238795325112867385, 1.000000000000000000, 0.9238795325112867385, 1.000000000000000000, 0.9238795325112867385, 1.000000000000000000, 0.9238795325112867385, 1.000000000000000000, 0.9238795325112867385, 1.000000000000000000, 0.9238795325112867385, 1.000000000000000000, 0.9238795325112867385, 1.000000000000000000, 0.9238795325112867385, 1.000000000000000000, 0.9238795325112867385, 1.000000000000000000, 0.9238795325112867385, 1.000000000000000000, 0.9238795325112867385, 1.000000000000000000, 0.9238795325112867385, 1.000000000000000000, 0.9238795325112867385, 1.000000000000000000, 0.9238795325112867385, 1.000000000000000000, 0.9238795325112867385, 1.000000000000000000, 0.9238795325112867385, 1.000000000000000000, 0.9238795325112867385, 1.000000000000000000) ) ) 
 REPRESENTATION_ITEM ( '' )  SURFACE ( )  );
#7754=CARTESIAN_POINT ( 'NONE',  ( 2.461020065508804144, 0.5233572909743210433, -2.501033807289417599 ) ) ;
#7764=CARTESIAN_POINT ( 'NONE',  ( 2.066987299999999639, 0.8561741729129456191, -2.099999998907525534 ) ) ;
#7766=( NAMED_UNIT ( * ) SI_UNIT ( $, .STERADIAN. ) SOLID_ANGLE_UNIT ( ) );
#7772=EDGE_CURVE ( 'NONE', #9805, #5611, #7686, .T. ) ;
#7773=CARTESIAN_POINT ( 'NONE',  ( -2.500000000000000000, -1.035533905932739307, -2.949999997815051067 ) ) ;
#7774=CARTESIAN_POINT ( 'NONE',  ( 3.796994071234844259E-16, -2.066987299999999639, 0.6500000010924747995 ) ) ;
#7795=ORIENTED_EDGE ( 'NONE', *, *, #10097, .F. ) ;
#7803=CARTESIAN_POINT ( 'NONE',  ( 1.035533905932737531, 2.500000000000000444, 1.550000002184949821 ) ) ;
#7808=CARTESIAN_POINT ( 'NONE',  ( 0.8561741729129451750, 2.066987299999999639, 0.4000000010924749105 ) ) ;
#7810=AXIS2_PLACEMENT_3D ( 'NONE', #12336, #10916, #3744 ) ;
#7812=VERTEX_POINT ( 'NONE', #15166 ) ;
#7818=CARTESIAN_POINT ( 'NONE',  ( -1.530808498934191571E-16, 2.500000000000000000, 1.600000002184949643 ) ) ;
#7834=CARTESIAN_POINT ( 'NONE',  ( 1.722248641545789605, -1.834520197013864484, -2.499366215161968885 ) ) ;
#7835=ORIENTED_EDGE ( 'NONE', *, *, #8923, .F. ) ;
#7846=CARTESIAN_POINT ( 'NONE',  ( -1.530808498934191571E-16, 2.500000000000000000, -0.1000000000000002554 ) ) ;
#7857=CARTESIAN_POINT ( 'NONE',  ( -0.8561741729129455081, 2.066987299999999639, -2.099999998907525089 ) ) ;
#7862=EDGE_CURVE ( 'NONE', #3215, #786, #15402, .T. ) ;
#7882=CARTESIAN_POINT ( 'NONE',  ( -1.530808498934191571E-16, 2.500000000000000000, -1.700000000000000622 ) ) ;
#7885=CARTESIAN_POINT ( 'NONE',  ( -2.500000000000000000, -0.9567085809127248153, 1.846193978810514169 ) ) ;
#7888=CARTESIAN_POINT ( 'NONE',  ( -1.530808498934191571E-16, 2.500000000000000000, -0.7999999978150504898 ) ) ;
#7890=CYLINDRICAL_SURFACE ( 'NONE', #3138, 2.500000000000000000 ) ;
#7899=CARTESIAN_POINT ( 'NONE',  ( -1.035533905932738197, -2.500000000000000000, 0.3500000021849494769 ) ) ;
#7909=CARTESIAN_POINT ( 'NONE',  ( 0.5843386044905307664, -2.435052651710797544, -2.500695021345132663 ) ) ;
#7919=CARTESIAN_POINT ( 'NONE',  ( 1.035533905932739085, -2.500000000000000000, -1.250000000000000222 ) ) ;
#7921=CARTESIAN_POINT ( 'NONE',  ( 2.500000000000000444, 1.035533905932737975, 1.450000002184949954 ) ) ;
#7926=CARTESIAN_POINT ( 'NONE',  ( -2.066987299999999639, 0.8561741729129455081, -1.199999998907525178 ) ) ;
#7935=( BOUNDED_CURVE ( )  B_SPLINE_CURVE ( 2, ( #8838, #5174, #11056, #8687, #7403, #7251, #13592 ),
 .UNSPECIFIED., .F., .F. ) 
 B_SPLINE_CURVE_WITH_KNOTS ( ( 3, 2, 2, 3 ),
 ( 0.7142857142857143016, 0.7321428571428570953, 0.7500000000000000000, 0.7678571432794594198 ),
 .UNSPECIFIED. ) 
 CURVE ( )  GEOMETRIC_REPRESENTATION_ITEM ( )  RATIONAL_B_SPLINE_CURVE ( ( 1.000000000000000000, 0.9238795325112867385, 1.000000000000000000, 0.9238795325112867385, 1.000000000000000000, 0.9238795325112867385, 1.000000000000000000 ) ) 
 REPRESENTATION_ITEM ( '' )  );
#7948=EDGE_LOOP ( 'NONE', ( #10767, #10418 ) ) ;
#7961=CARTESIAN_POINT ( 'NONE',  ( 2.999999999999999556, -1.732050807568877859, -2.500000000000000000 ) ) ;
#7962=CARTESIAN_POINT ( 'NONE',  ( 4.592425496802573972E-16, -2.500000000000000000, -1.300000000000000044 ) ) ;
#7963=CARTESIAN_POINT ( 'NONE',  ( 1.035533905932739085, -2.500000000000000000, -1.250000000000000222 ) ) ;
#7968=VERTEX_POINT ( 'NONE', #11967 ) ;
#7976=CARTESIAN_POINT ( 'NONE',  ( 2.500000000000000444, -1.035533905932737309, 1.350000002184949421 ) ) ;
#7984=CARTESIAN_POINT ( 'NONE',  ( 3.796994071234844259E-16, -2.066987299999999639, 0.6500000010924747995 ) ) ;
#7987=ADVANCED_FACE ( 'NONE', ( #14434 ), #2023, .F. ) ;
#7994=FACE_OUTER_BOUND ( 'NONE', #10842, .T. ) ;
#7999=CARTESIAN_POINT ( 'NONE',  ( -1.035533905932737753, 2.500000000000000444, -1.649999999999999911 ) ) ;
#8000=DIRECTION ( 'NONE',  ( 0.000000000000000000, -1.000000000000000000, 0.000000000000000000 ) ) ;
#8010=CARTESIAN_POINT ( 'NONE',  ( -2.066987299999999639, 0.000000000000000000, -1.149999998907525356 ) ) ;
#8013=CARTESIAN_POINT ( 'NONE',  ( -1.035533905932737753, 2.500000000000000444, -1.549999997815050268 ) ) ;
#8021=CARTESIAN_POINT ( 'NONE',  ( 2.500000000000000444, -1.035533905932737309, -0.2499999978150503066 ) ) ;
#8034=( BOUNDED_CURVE ( )  B_SPLINE_CURVE ( 2, ( #11640, #2011, #14252, #14178, #743, #2161, #5608, #3360, #6884 ),
 .UNSPECIFIED., .F., .F. ) 
 B_SPLINE_CURVE_WITH_KNOTS ( ( 3, 2, 2, 2, 3 ),
 ( 0.1428571428571428492, 0.1607142857142857262, 0.1785714285714285754, 0.1964285714285714246, 0.2142857142857142738 ),
 .UNSPECIFIED. ) 
 CURVE ( )  GEOMETRIC_REPRESENTATION_ITEM ( )  RATIONAL_B_SPLINE_CURVE ( ( 1.000000000000000000, 0.9238795325112867385, 1.000000000000000000, 0.9238795325112867385, 1.000000000000000000, 0.9238795325112867385, 1.000000000000000000, 0.9238795325112867385, 1.000000000000000000 ) ) 
 REPRESENTATION_ITEM ( '' )  );
#8038=CARTESIAN_POINT ( 'NONE',  ( -1.530808498934191571E-16, 2.500000000000000000, 2.184949703804006660E-09 ) ) ;
#8042=CARTESIAN_POINT ( 'NONE',  ( 2.500000000000000444, -1.035533905932737309, -1.049999997815050268 ) ) ;
#8045=CARTESIAN_POINT ( 'NONE',  ( 1.767766952966368654, 1.767766952966369098, -0.8999999978150502455 ) ) ;
#8046=CARTESIAN_POINT ( 'NONE',  ( -2.066987299999999639, 0.000000000000000000, -2.549999998907525711 ) ) ;
#8057=CARTESIAN_POINT ( 'NONE',  ( -1.035533905932737753, 2.500000000000000444, -0.7499999978150505564 ) ) ;
#8059=CARTESIAN_POINT ( 'NONE',  ( 1.500000000000000000, 1.836970198721029934E-16, 2.500000000000000000 ) ) ;
#8061=CARTESIAN_POINT ( 'NONE',  ( -2.500000000000000444, 1.035533905932737753, 2.456999999978150662 ) ) ;
#8075=CARTESIAN_POINT ( 'NONE',  ( -3.000000000000000000, 1.732050807568877415, -5.500000000000000000 ) ) ;
#8080=CARTESIAN_POINT ( 'NONE',  ( 1.536366799937288086, 1.999167105995449445, -2.499999999999999556 ) ) ;
#8082=CARTESIAN_POINT ( 'NONE',  ( 1.035533905932737531, 2.500000000000000444, -0.1499999999999999667 ) ) ;
#8089=DIRECTION ( 'NONE',  ( 0.000000000000000000, 0.000000000000000000, 1.000000000000000000 ) ) ;
#8093=CARTESIAN_POINT ( 'NONE',  ( -2.066987299999999639, 0.000000000000000000, -0.3499999989075254225 ) ) ;
#8098=CARTESIAN_POINT ( 'NONE',  ( -2.500000000000000000, 0.000000000000000000, -1.399999997815050357 ) ) ;
#8101=CARTESIAN_POINT ( 'NONE',  ( -1.084202172485504434E-16, 3.464101615137754830, -5.500000000000000000 ) ) ;
#8122=CARTESIAN_POINT ( 'NONE',  ( -1.035533905932738197, -2.500000000000000000, 0.3500000021849497545 ) ) ;
#8135=CARTESIAN_POINT ( 'NONE',  ( 1.767766952966369320, -1.767766952966368654, -1.099999997815050534 ) ) ;
#8137=EDGE_CURVE ( 'NONE', #13466, #4492, #7438, .T. ) ;
#8142=CARTESIAN_POINT ( 'NONE',  ( 1.035533905932739085, -2.500000000000000000, 1.156999999978150395 ) ) ;
#8146=CARTESIAN_POINT ( 'NONE',  ( -2.066987299999999639, 0.8561741729129452860, 2.000000001092474555 ) ) ;
#8161=CARTESIAN_POINT ( 'NONE',  ( 1.767766952966368654, 1.767766952966369098, -1.000000000000000000 ) ) ;
#8170=CARTESIAN_POINT ( 'NONE',  ( -0.8561741729129458411, -2.066987299999999195, -0.9999999989075253337 ) ) ;
#8174=CARTESIAN_POINT ( 'NONE',  ( 0.000000000000000000, 0.000000000000000000, 2.500000000000000000 ) ) ;
#8185=DIRECTION ( 'NONE',  ( 0.000000000000000000, 0.000000000000000000, -1.000000000000000000 ) ) ;
#8196=ORIENTED_EDGE ( 'NONE', *, *, #10028, .F. ) ;
#8203=CARTESIAN_POINT ( 'NONE',  ( -2.500000000000000444, 1.035533905932737753, 0.1500000021849498544 ) ) ;
#8207=CARTESIAN_POINT ( 'NONE',  ( 2.066987299999999639, 0.8561741729129456191, -2.099999998907525534 ) ) ;
#8216=CARTESIAN_POINT ( 'NONE',  ( 1.767766952966368654, 1.767766952966369098, -2.499999997815050445 ) ) ;
#8221=CARTESIAN_POINT ( 'NONE',  ( -2.500000000000000000, -1.035533905932739307, 0.9569999999781505506 ) ) ;
#8225=CARTESIAN_POINT ( 'NONE',  ( -2.066987299999999195, -0.8561741729129466183, -0.2999999989075253226 ) ) ;
#8229=ORIENTED_EDGE ( 'NONE', *, *, #8923, .T. ) ;
#8239=DIRECTION ( 'NONE',  ( 0.000000000000000000, 0.000000000000000000, -1.000000000000000000 ) ) ;
#8252=CARTESIAN_POINT ( 'NONE',  ( -1.084202172485504434E-15, -3.464101615137755275, -2.500000000000000000 ) ) ;
#8263=DIRECTION ( 'NONE',  ( -1.000000000000000000, 0.000000000000000000, 0.000000000000000000 ) ) ;
#8267=CARTESIAN_POINT ( 'NONE',  ( -1.461580736456472351, -1.461580736456473018, -0.8499999989075254225 ) ) ;
#8282=CARTESIAN_POINT ( 'NONE',  ( 2.500000000000000000, 3.061616997868383141E-16, -0.9999999978150501123 ) ) ;
#8295=CARTESIAN_POINT ( 'NONE',  ( -1.035533905932737753, 2.500000000000000444, -2.349999997815050090 ) ) ;
#8299=CARTESIAN_POINT ( 'NONE',  ( 4.592425496802573972E-16, -2.500000000000000000, 1.106999999978150573 ) ) ;
#8301=CARTESIAN_POINT ( 'NONE',  ( 0.8561741729129451750, 2.066987299999999639, 1.800000001092475266 ) ) ;
#8308=DIRECTION ( 'NONE',  ( 0.000000000000000000, 0.000000000000000000, -1.000000000000000000 ) ) ;
#8319=CARTESIAN_POINT ( 'NONE',  ( 1.035533905932739085, -2.500000000000000000, -1.149999997815050135 ) ) ;
#8329=EDGE_LOOP ( 'NONE', ( #9321, #6867 ) ) ;
#8335=FACE_OUTER_BOUND ( 'NONE', #1351, .T. ) ;
#8340=CARTESIAN_POINT ( 'NONE',  ( -2.066987299999999195, -0.8561741729129466183, 0.7000000010924749549 ) ) ;
#8349=CARTESIAN_POINT ( 'NONE',  ( -2.066987299999999639, 0.8561741729129455081, 1.400000001092474911 ) ) ;
#8350=CARTESIAN_POINT ( 'NONE',  ( 1.767766952966368654, 1.767766952966369098, 1.399999999999999911 ) ) ;
#8366=CARTESIAN_POINT ( 'NONE',  ( -2.500000000000000000, 0.000000000000000000, -1.399999997815050357 ) ) ;
#8370=CARTESIAN_POINT ( 'NONE',  ( -2.500000000000000000, -1.035533905932739307, 0.9499999999999999556 ) ) ;
#8380=CARTESIAN_POINT ( 'NONE',  ( 1.035533905932737531, 2.500000000000000444, -1.649999997815050579 ) ) ;
#8382=CARTESIAN_POINT ( 'NONE',  ( -1.035533905932737753, 2.500000000000000444, -0.05000000000000013461 ) ) ;
#8385=CARTESIAN_POINT ( 'NONE',  ( -1.767766952966368432, -1.767766952966369320, -1.393000000021849649 ) ) ;
#8386=CARTESIAN_POINT ( 'NONE',  ( -2.066987299999999639, 0.000000000000000000, 2.050000001092474822 ) ) ;
#8388=CARTESIAN_POINT ( 'NONE',  ( 3.796994071234844259E-16, -2.066987299999999639, -0.9499999989075252893 ) ) ;
#8392=AXIS2_PLACEMENT_3D ( 'NONE', #8562, #1219, #3530 ) ;
#8401=CARTESIAN_POINT ( 'NONE',  ( 2.500000000000000000, 3.061616997868383141E-16, 2.500000000000000000 ) ) ;
#8402=AXIS2_PLACEMENT_3D ( 'NONE', #3876, #3803, #13436 ) ;
#8423=CARTESIAN_POINT ( 'NONE',  ( 0.8561741729129463963, -2.066987299999999195, -0.6999999989075250673 ) ) ;
#8430=CARTESIAN_POINT ( 'NONE',  ( -2.066987299999999639, 0.8561741729129455081, -0.1999999989075250117 ) ) ;
#8437=PLANE ( 'NONE',  #13146 ) ;
#8446=AXIS2_PLACEMENT_3D ( 'NONE', #1223, #2257, #12046 ) ;
#8447=CARTESIAN_POINT ( 'NONE',  ( -1.767766952966369098, 1.767766952966369098, -3.099999997815050090 ) ) ;
#8455=VERTEX_POINT ( 'NONE', #8386 ) ;
#8462=CARTESIAN_POINT ( 'NONE',  ( 2.500000000000000444, -1.035533905932737309, -1.849999997815050534 ) ) ;
#8466=CARTESIAN_POINT ( 'NONE',  ( -2.500000000000000444, 1.035533905932737753, 0.8500000000000001998 ) ) ;
#8471=CARTESIAN_POINT ( 'NONE',  ( -2.066987299999999195, -0.8561741729129466183, 1.500000001092474777 ) ) ;
#8479=CARTESIAN_POINT ( 'NONE',  ( 0.000000000000000000, 0.000000000000000000, 2.500000000000000000 ) ) ;
#8505=CYLINDRICAL_SURFACE ( 'NONE', #3837, 2.500000000000000000 ) ;
#8507=CARTESIAN_POINT ( 'NONE',  ( -0.8561741729129458411, -2.066987299999999195, 1.600000001092474866 ) ) ;
#8513=CARTESIAN_POINT ( 'NONE',  ( 0.8561741729129452860, 2.066987299999999639, 1.200000001092474733 ) ) ;
#8521=SURFACE_STYLE_USAGE ( .BOTH. , #10970 ) ;
#8524=CARTESIAN_POINT ( 'NONE',  ( 2.500000000000000000, 3.061616997868383141E-16, 2.500000000000000000 ) ) ;
#8529=CARTESIAN_POINT ( 'NONE',  ( -1.035533905932738197, -2.500000000000000000, -2.849999997815050978 ) ) ;
#8541=CARTESIAN_POINT ( 'NONE',  ( 2.500000000000000444, -1.035533905932737309, -2.649999997815050357 ) ) ;
#8546=CARTESIAN_POINT ( 'NONE',  ( 2.500000000000000000, 3.061616997868383141E-16, -0.2999999999999999334 ) ) ;
#8548=CARTESIAN_POINT ( 'NONE',  ( 2.500000000000000444, -1.035533905932737309, 2.049999999999999822 ) ) ;
#8553=CARTESIAN_POINT ( 'NONE',  ( -0.8561741729129455081, 2.066987299999999639, 2.100000001092475088 ) ) ;
#8554=CARTESIAN_POINT ( 'NONE',  ( -1.035533905932737753, 2.500000000000000444, -2.450000000000000178 ) ) ;
#8556=CARTESIAN_POINT ( 'NONE',  ( 0.000000000000000000, 0.000000000000000000, 2.500000000000000000 ) ) ;
#8560=ORIENTED_EDGE ( 'NONE', *, *, #11808, .T. ) ;
#8562=CARTESIAN_POINT ( 'NONE',  ( -1.084202172485504434E-15, -3.464101615137755275, -5.500000000000000000 ) ) ;
#8579=VECTOR ( 'NONE', #2457, 1000.000000000000000 ) ;
#8580=CARTESIAN_POINT ( 'NONE',  ( 0.000000000000000000, 0.000000000000000000, 2.500000000000000000 ) ) ;
#8581=CARTESIAN_POINT ( 'NONE',  ( 2.500000000000000444, 1.035533905932737975, -1.050000000000000044 ) ) ;
#8585=CARTESIAN_POINT ( 'NONE',  ( 0.8561741729129451750, 2.066987299999999639, 0.4000000010924749105 ) ) ;
#8592=CARTESIAN_POINT ( 'NONE',  ( -2.066987299999999195, -0.8561741729129467293, 0.7000000010924749549 ) ) ;
#8594=CARTESIAN_POINT ( 'NONE',  ( -1.530808498934191571E-16, 2.500000000000000000, 1.500000000000000000 ) ) ;
#8620=CARTESIAN_POINT ( 'NONE',  ( -2.066987299999999195, -0.8561741729129466183, -0.2999999989075253226 ) ) ;
#8622=CARTESIAN_POINT ( 'NONE',  ( -1.767766952966369098, 1.767766952966369098, 0.000000000000000000 ) ) ;
#8624=CARTESIAN_POINT ( 'NONE',  ( 2.500000000000000444, 1.035533905932737975, 0.5499999999999999334 ) ) ;
#8628=CARTESIAN_POINT ( 'NONE',  ( -1.461580736456472795, 1.461580736456472795, -1.249999998907525223 ) ) ;
#8648=CARTESIAN_POINT ( 'NONE',  ( -2.500000000000000000, 0.000000000000000000, 2.500000000000000000 ) ) ;
#8654=ORIENTED_EDGE ( 'NONE', *, *, #12700, .F. ) ;
#8658=CARTESIAN_POINT ( 'NONE',  ( 2.500000000000000000, 3.061616997868383141E-16, 1.300000000000000044 ) ) ;
#8661=CARTESIAN_POINT ( 'NONE',  ( -2.066987299999999195, -0.8561741729129466183, 1.500000001092474777 ) ) ;
#8663=LINE ( 'NONE', #9927, #13821 ) ;
#8665=CARTESIAN_POINT ( 'NONE',  ( -1.767766952966368432, -1.767766952966369320, -0.6000000000000003109 ) ) ;
#8667=FACE_OUTER_BOUND ( 'NONE', #9787, .T. ) ;
#8683=CARTESIAN_POINT ( 'NONE',  ( 1.767766952966369320, -1.767766952966368654, -1.899999997815050357 ) ) ;
#8687=CARTESIAN_POINT ( 'NONE',  ( -1.035533905932737753, 2.500000000000000444, -2.349999997815050090 ) ) ;
#8696=CARTESIAN_POINT ( 'NONE',  ( 1.461580736456472573, 1.461580736456472795, -1.449999998907525178 ) ) ;
#8700=CARTESIAN_POINT ( 'NONE',  ( -1.035533905932737753, 2.500000000000000444, 0.7500000000000001110 ) ) ;
#8703=CARTESIAN_POINT ( 'NONE',  ( 0.8561741729129451750, 2.066987299999999639, -2.199999998907525622 ) ) ;
#8706=ORIENTED_EDGE ( 'NONE', *, *, #7371, .F. ) ;
#8726=CARTESIAN_POINT ( 'NONE',  ( -0.2790400018234628354, 2.500000000000000444, -2.501110090150877152 ) ) ;
#8734=CARTESIAN_POINT ( 'NONE',  ( -2.500000000000000000, 0.000000000000000000, 1.700000000000000178 ) ) ;
#8739=CARTESIAN_POINT ( 'NONE',  ( 1.035533905932739085, -2.500000000000000000, -0.4499999999999999556 ) ) ;
#8744=CARTESIAN_POINT ( 'NONE',  ( 2.066987300000000083, -0.8561741729129450640, 0.8000000010924748217 ) ) ;
#8772=CARTESIAN_POINT ( 'NONE',  ( 1.461580736456473018, -1.461580736456472573, -1.649999998907525356 ) ) ;
#8776=CARTESIAN_POINT ( 'NONE',  ( -2.500000000000000000, 0.000000000000000000, 1.700000000000000178 ) ) ;
#8781=CARTESIAN_POINT ( 'NONE',  ( -2.066987299999999639, 0.8561741729129452860, -0.9999999989075254447 ) ) ;
#8784=VERTEX_POINT ( 'NONE', #15442 ) ;
#8813=CARTESIAN_POINT ( 'NONE',  ( 1.767766952966368654, 1.767766952966369098, 2.200000000000000178 ) ) ;
#8819=CARTESIAN_POINT ( 'NONE',  ( 3.796994071234844259E-16, -2.066987299999999639, -1.549999998907525045 ) ) ;
#8823=CARTESIAN_POINT ( 'NONE',  ( -0.8561741729129455081, 2.066987299999999639, 0.3000000010924747662 ) ) ;
#8838=CARTESIAN_POINT ( 'NONE',  ( -2.500000000000000000, 0.000000000000000000, -2.199999997815050623 ) ) ;
#8851=CARTESIAN_POINT ( 'NONE',  ( -0.8561741729129455081, 2.066987299999999639, -2.099999998907525089 ) ) ;
#8856=CARTESIAN_POINT ( 'NONE',  ( -1.530808498934191571E-16, 2.500000000000000000, -0.9000000000000002442 ) ) ;
#8861=CARTESIAN_POINT ( 'NONE',  ( -2.066987299999999639, 0.000000000000000000, -0.1499999989075253282 ) ) ;
#8869=VECTOR ( 'NONE', #11567, 1000.000000000000227 ) ;
#8884=AXIS2_PLACEMENT_3D ( 'NONE', #10308, #15316, #15396 ) ;
#8896=CARTESIAN_POINT ( 'NONE',  ( -1.461580736456472795, 1.461580736456472795, -1.849999998907525534 ) ) ;
#8903=CARTESIAN_POINT ( 'NONE',  ( 2.066987299999999639, 2.531329380823229670E-16, -1.349999998907525534 ) ) ;
#8923=EDGE_CURVE ( 'NONE', #13408, #5765, #3497, .T. ) ;
#8924=ORIENTED_EDGE ( 'NONE', *, *, #9799, .T. ) ;
#8929=EDGE_LOOP ( 'NONE', ( #2050, #15140, #9478, #15472 ) ) ;
#8930=CARTESIAN_POINT ( 'NONE',  ( 3.796994071234844259E-16, -2.066987299999999639, -1.749999998907525223 ) ) ;
#8934=CARTESIAN_POINT ( 'NONE',  ( -2.500000000000000000, 0.000000000000000000, -0.7000000000000000666 ) ) ;
#8938=CARTESIAN_POINT ( 'NONE',  ( 2.500000000000000444, 1.035533905932737975, -0.9499999978150504010 ) ) ;
#8939=CARTESIAN_POINT ( 'NONE',  ( 2.066987299999999639, 0.8561741729129456191, 0.3000000010924747662 ) ) ;
#8941=FACE_OUTER_BOUND ( 'NONE', #7659, .T. ) ;
#8942=EDGE_CURVE ( 'NONE', #5900, #8784, #12009, .T. ) ;
#8954=CARTESIAN_POINT ( 'NONE',  ( -2.500000000000000000, -1.035533905932739307, -2.250000000000000888 ) ) ;
#8956=CARTESIAN_POINT ( 'NONE',  ( 2.500000000000000444, -1.035533905932737309, 1.256999999978150706 ) ) ;
#8964=CARTESIAN_POINT ( 'NONE',  ( 0.4428048500434558221, -2.464588252924116318, -2.500827920915885461 ) ) ;
#8966=ORIENTED_EDGE ( 'NONE', *, *, #12512, .F. ) ;
#8975=CARTESIAN_POINT ( 'NONE',  ( -2.066987299999999639, 0.000000000000000000, -2.549999998907525711 ) ) ;
#8981=CARTESIAN_POINT ( 'NONE',  ( -1.265664690411614835E-16, 2.066987299999999639, -2.749999998907525001 ) ) ;
#8985=CARTESIAN_POINT ( 'NONE',  ( 3.796994071234844259E-16, -2.066987299999999639, 1.450000001092474733 ) ) ;
#8991=( BOUNDED_SURFACE ( )  B_SPLINE_SURFACE ( 1, 2, ( 
 ( #5444, #15217, #2969, #15455, #7818, #4400, #14017, #6641, #9326, #7976, #2076, #12973, #9254, #6949, #6717, #12740, #13857, #12669, #10522, #14168, #11781, #3123, #14088, #5518, #808, #10366, #1842, #575, #646, #7899, #11549, #4317, #5598, #730, #1766, #9178, #12816, #15376, #1998, #4238, #11628, #10444, #1921, #11471, #3273, #6794, #4472, #883, #15298, #3199, #9106, #8057, #10289, #5751, #6873, #11707, #5674, #15142, #8135, #13935, #10595, #14317, #11939, #7101, #7025, #1045, #3588, #88, #12180, #8380, #15691, #10753, #14240, #8462, #5830, #10991, #3424, #5908, #15612, #11853, #4713, #13296, #3667, #8295, #12098, #3350, #8216, #2232, #1278, #8541, #13369, #2312, #5987, #13218, #4795, #13132, #10830, #9564, #1197, #14404, #9486 ),
 ( #9650, #4631, #13052, #2393, #6152, #3511, #2478, #9732, #9404, #964, #7338, #7261, #2150, #14491, #10675, #6071, #10915, #7184, #13, #12022, #1122, #15535, #4875, #14570, #12570, #2558, #14656, #14812, #11146, #5185, #5269, #3743, #6389, #325, #1356, #11066, #1668, #13529, #9961, #13763, #6469, #6308, #3975, #2872, #248, #9883, #167, #8620, #3823, #14736, #7489, #12334, #11223, #11377, #7415, #5028, #10116, #12415, #6231, #4956, #10039, #1513, #13455, #6544, #7720, #9806, #7644, #2635, #5108, #1431, #8696, #3897, #4060, #2715, #8772, #13684, #8930, #11302, #12257, #13603, #14969, #7567, #14888, #8851, #12491, #1591, #2794, #399, #5425, #480, #6622, #1747, #1825, #707, #15576, #13915, #11454, #6698, #11900, #4219, #9234 ) ),
 .UNSPECIFIED., .F., .F., .F. ) 
 B_SPLINE_SURFACE_WITH_KNOTS ( ( 2, 2 ),
 ( 3, 2, 2, 2, 2, 2, 2, 2, 2, 2, 2, 2, 2, 2, 2, 2, 2, 2, 2, 2, 2, 2, 2, 2, 2, 2, 2, 2, 2, 2, 2, 2, 2, 2, 2, 2, 2, 2, 2, 2, 2, 2, 2, 2, 2, 2, 2, 2, 2, 2, 3 ),
 ( 0.000000000000000000, 1.000000000000000000 ),
 ( 0.000000000000000000, 0.01785714285714285615, 0.03571428571428571230, 0.05357142857142856845, 0.07142857142857142461, 0.08928571428571428770, 0.1071428571428571369, 0.1250000000000000000, 0.1428571428571428492, 0.1607142857142857262, 0.1785714285714285754, 0.1964285714285714246, 0.2142857142857142738, 0.2321428571428571508, 0.2500000000000000000, 0.2678571428571428492, 0.2857142857142856984, 0.3035714285714285476, 0.3214285714285714524, 0.3392857142857143016, 0.3571428571428571508, 0.3750000000000000000, 0.3928571428571428492, 0.4107142857142856984, 0.4285714285714285476, 0.4464285714285714524, 0.4642857142857143016, 0.4821428571428571508, 0.5000000000000000000, 0.5178571428571429047, 0.5357142857142856984, 0.5535714285714286031, 0.5714285714285713969, 0.5892857142857143016, 0.6071428571428570953, 0.6250000000000000000, 0.6428571428571429047, 0.6607142857142856984, 0.6785714285714286031, 0.6964285714285713969, 0.7142857142857143016, 0.7321428571428570953, 0.7500000000000000000, 0.7678571428571429047, 0.7857142857142856984, 0.8035714285714286031, 0.8214285714285713969, 0.8392857142857143016, 0.8571428571428570953, 0.8750000000000000000, 0.8928571428571429047 ),
 .UNSPECIFIED. ) 
 GEOMETRIC_REPRESENTATION_ITEM ( )  RATIONAL_B_SPLINE_SURFACE ( (
 ( 1.000000000000000000, 0.9238795325112867385, 1.000000000000000000, 0.9238795325112867385, 1.000000000000000000, 0.9238795325112867385, 1.000000000000000000, 0.9238795325112867385, 1.000000000000000000, 0.9238795325112867385, 1.000000000000000000, 0.9238795325112867385, 1.000000000000000000, 0.9238795325112867385, 1.000000000000000000, 0.9238795325112867385, 1.000000000000000000, 0.9238795325112867385, 1.000000000000000000, 0.9238795325112867385, 1.000000000000000000, 0.9238795325112867385, 1.000000000000000000, 0.9238795325112867385, 1.000000000000000000, 0.9238795325112867385, 1.000000000000000000, 0.9238795325112867385, 1.000000000000000000, 0.9238795325112867385, 1.000000000000000000, 0.9238795325112867385, 1.000000000000000000, 0.9238795325112867385, 1.000000000000000000, 0.9238795325112867385, 1.000000000000000000, 0.9238795325112867385, 1.000000000000000000, 0.9238795325112867385, 1.000000000000000000, 0.9238795325112867385, 1.000000000000000000, 0.9238795325112867385, 1.000000000000000000, 0.9238795325112867385, 1.000000000000000000, 0.9238795325112867385, 1.000000000000000000, 0.9238795325112867385, 1.000000000000000000, 0.9238795325112867385, 1.000000000000000000, 0.9238795325112867385, 1.000000000000000000, 0.9238795325112867385, 1.000000000000000000, 0.9238795325112867385, 1.000000000000000000, 0.9238795325112867385, 1.000000000000000000, 0.9238795325112867385, 1.000000000000000000, 0.9238795325112867385, 1.000000000000000000, 0.9238795325112867385, 1.000000000000000000, 0.9238795325112867385, 1.000000000000000000, 0.9238795325112867385, 1.000000000000000000, 0.9238795325112867385, 1.000000000000000000, 0.9238795325112867385, 1.000000000000000000, 0.9238795325112867385, 1.000000000000000000, 0.9238795325112867385, 1.000000000000000000, 0.9238795325112867385, 1.000000000000000000, 0.9238795325112867385, 1.000000000000000000, 0.9238795325112867385, 1.000000000000000000, 0.9238795325112867385, 1.000000000000000000, 0.9238795325112867385, 1.000000000000000000, 0.9238795325112867385, 1.000000000000000000, 0.9238795325112867385, 1.000000000000000000, 0.9238795325112867385, 1.000000000000000000, 0.9238795325112867385, 1.000000000000000000, 0.9238795325112867385, 1.000000000000000000, 0.9238795325112867385, 1.000000000000000000),
 ( 1.000000000000000000, 0.9238795325112867385, 1.000000000000000000, 0.9238795325112867385, 1.000000000000000000, 0.9238795325112867385, 1.000000000000000000, 0.9238795325112867385, 1.000000000000000000, 0.9238795325112867385, 1.000000000000000000, 0.9238795325112867385, 1.000000000000000000, 0.9238795325112867385, 1.000000000000000000, 0.9238795325112867385, 1.000000000000000000, 0.9238795325112867385, 1.000000000000000000, 0.9238795325112867385, 1.000000000000000000, 0.9238795325112867385, 1.000000000000000000, 0.9238795325112867385, 1.000000000000000000, 0.9238795325112867385, 1.000000000000000000, 0.9238795325112867385, 1.000000000000000000, 0.9238795325112867385, 1.000000000000000000, 0.9238795325112867385, 1.000000000000000000, 0.9238795325112867385, 1.000000000000000000, 0.9238795325112867385, 1.000000000000000000, 0.9238795325112867385, 1.000000000000000000, 0.9238795325112867385, 1.000000000000000000, 0.9238795325112867385, 1.000000000000000000, 0.9238795325112867385, 1.000000000000000000, 0.9238795325112867385, 1.000000000000000000, 0.9238795325112867385, 1.000000000000000000, 0.9238795325112867385, 1.000000000000000000, 0.9238795325112867385, 1.000000000000000000, 0.9238795325112867385, 1.000000000000000000, 0.9238795325112867385, 1.000000000000000000, 0.9238795325112867385, 1.000000000000000000, 0.9238795325112867385, 1.000000000000000000, 0.9238795325112867385, 1.000000000000000000, 0.9238795325112867385, 1.000000000000000000, 0.9238795325112867385, 1.000000000000000000, 0.9238795325112867385, 1.000000000000000000, 0.9238795325112867385, 1.000000000000000000, 0.9238795325112867385, 1.000000000000000000, 0.9238795325112867385, 1.000000000000000000, 0.9238795325112867385, 1.000000000000000000, 0.9238795325112867385, 1.000000000000000000, 0.9238795325112867385, 1.000000000000000000, 0.9238795325112867385, 1.000000000000000000, 0.9238795325112867385, 1.000000000000000000, 0.9238795325112867385, 1.000000000000000000, 0.9238795325112867385, 1.000000000000000000, 0.9238795325112867385, 1.000000000000000000, 0.9238795325112867385, 1.000000000000000000, 0.9238795325112867385, 1.000000000000000000, 0.9238795325112867385, 1.000000000000000000, 0.9238795325112867385, 1.000000000000000000, 0.9238795325112867385, 1.000000000000000000) ) ) 
 REPRESENTATION_ITEM ( '' )  SURFACE ( )  );
#9011=LINE ( 'NONE', #556, #1057 ) ;
#9014=CARTESIAN_POINT ( 'NONE',  ( 1.035533905932739085, -2.500000000000000000, -2.049999999999999822 ) ) ;
#9020=CARTESIAN_POINT ( 'NONE',  ( -2.066987299999999195, -0.8561741729129466183, -0.09999999890752520049 ) ) ;
#9022=AXIS2_PLACEMENT_3D ( 'NONE', #6901, #11732, #6821 ) ;
#9023=ORIENTED_EDGE ( 'NONE', *, *, #5808, .T. ) ;
#9054=CARTESIAN_POINT ( 'NONE',  ( -1.461580736456472351, -1.461580736456473018, -1.649999998907525356 ) ) ;
#9056=( LENGTH_UNIT ( ) NAMED_UNIT ( * ) SI_UNIT ( .MILLI., .METRE. ) );
#9062=CARTESIAN_POINT ( 'NONE',  ( 3.796994071234844259E-16, -2.066987299999999639, -0.1499999989075253282 ) ) ;
#9063=ADVANCED_FACE ( 'NONE', ( #8941 ), #7890, .T. ) ;
#9072=CARTESIAN_POINT ( 'NONE',  ( 0.000000000000000000, 0.000000000000000000, 2.500000000000000000 ) ) ;
#9091=CARTESIAN_POINT ( 'NONE',  ( -1.035533905932738197, -2.500000000000000000, -0.5500000000000001554 ) ) ;
#9095=CARTESIAN_POINT ( 'NONE',  ( -0.8561741729129455081, 2.066987299999999639, -1.899999998907525134 ) ) ;
#9106=CARTESIAN_POINT ( 'NONE',  ( -1.767766952966369098, 1.767766952966369098, -0.6999999978150504010 ) ) ;
#9120=CARTESIAN_POINT ( 'NONE',  ( 0.1601274832639230095, -2.498925885410993697, -2.500580210930910319 ) ) ;
#9130=CARTESIAN_POINT ( 'NONE',  ( 2.500000000000000444, 1.035533905932737975, -1.050000000000000044 ) ) ;
#9137=CARTESIAN_POINT ( 'NONE',  ( -1.461580736456472351, -1.461580736456473018, -1.849999998907525534 ) ) ;
#9162=CARTESIAN_POINT ( 'NONE',  ( -2.500000000000000444, 1.035533905932737753, -1.549999999999999822 ) ) ;
#9165=CARTESIAN_POINT ( 'NONE',  ( 2.500000000000000444, -1.035533905932737309, -1.150000000000000133 ) ) ;
#9166=CARTESIAN_POINT ( 'NONE',  ( -2.500000000000000000, -1.035533905932739307, -1.450000000000000400 ) ) ;
#9169=LINE ( 'NONE', #10663, #413 ) ;
#9178=CARTESIAN_POINT ( 'NONE',  ( -1.035533905932737753, 2.500000000000000444, 0.05000000218494961984 ) ) ;
#9185=CARTESIAN_POINT ( 'NONE',  ( -1.461580736456472795, 1.461580736456472795, 1.950000001092474733 ) ) ;
#9189=ORIENTED_EDGE ( 'NONE', *, *, #1274, .T. ) ;
#9190=CARTESIAN_POINT ( 'NONE',  ( 1.965078059614901340, 1.570455839174875301, -2.498889909998655678 ) ) ;
#9195=ORIENTED_EDGE ( 'NONE', *, *, #4632, .F. ) ;
#9199=CARTESIAN_POINT ( 'NONE',  ( -1.530808498934191571E-16, 2.500000000000000000, -0.9000000000000002442 ) ) ;
#9201=CARTESIAN_POINT ( 'NONE',  ( -1.035533905932737753, 2.500000000000000444, 1.650000002184949910 ) ) ;
#9210=CARTESIAN_POINT ( 'NONE',  ( -0.8561741729129458411, -2.066987299999999195, -2.599999998907525534 ) ) ;
#9234=CARTESIAN_POINT ( 'NONE',  ( -1.265664690411614835E-16, 2.066987299999999639, -2.949999998907525178 ) ) ;
#9239=CARTESIAN_POINT ( 'NONE',  ( 1.035533905932739085, -2.500000000000000000, 0.4500000021849498988 ) ) ;
#9254=CARTESIAN_POINT ( 'NONE',  ( 4.592425496802573972E-16, -2.500000000000000000, 1.200000002184949510 ) ) ;
#9261=CARTESIAN_POINT ( 'NONE',  ( 2.066987299999999639, 2.531329380823229670E-16, 0.05000000109247476621 ) ) ;
#9267=CARTESIAN_POINT ( 'NONE',  ( -2.432277057295939571, -0.6446960933136758332, -2.500850192709198616 ) ) ;
#9270=VECTOR ( 'NONE', #4725, 1000.000000000000000 ) ;
#9276=CARTESIAN_POINT ( 'NONE',  ( 4.592425496802573972E-16, -2.500000000000000000, 1.899999999999999911 ) ) ;
#9277=CARTESIAN_POINT ( 'NONE',  ( 2.500000000000000000, 3.061616997868383141E-16, -1.100000000000000311 ) ) ;
#9279=FILL_AREA_STYLE_COLOUR ( '', #1768 ) ;
#9286=CARTESIAN_POINT ( 'NONE',  ( -2.066987299999999639, 0.000000000000000000, -1.949999998907525178 ) ) ;
#9299=DIRECTION ( 'NONE',  ( 0.000000000000000000, 0.000000000000000000, -1.000000000000000000 ) ) ;
#9302=VERTEX_POINT ( 'NONE', #7331 ) ;
#9309=CARTESIAN_POINT ( 'NONE',  ( 1.767766952966368654, 1.767766952966369098, -0.09999999781505011787 ) ) ;
#9313=CARTESIAN_POINT ( 'NONE',  ( 2.500000000000000444, 1.035533905932737975, -0.1499999978150502733 ) ) ;
#9321=ORIENTED_EDGE ( 'NONE', *, *, #9761, .F. ) ;
#9326=CARTESIAN_POINT ( 'NONE',  ( 2.500000000000000000, 3.061616997868383141E-16, 1.400000002184949688 ) ) ;
#9330=CARTESIAN_POINT ( 'NONE',  ( 1.767766952966368654, 1.767766952966369098, -0.9930000000218494050 ) ) ;
#9334=CARTESIAN_POINT ( 'NONE',  ( -1.461580736456472795, 1.461580736456472795, 1.150000001092474688 ) ) ;
#9342=EDGE_LOOP ( 'NONE', ( #2905, #1191, #15290, #14530 ) ) ;
#9346=EDGE_CURVE ( 'NONE', #10381, #546, #3389, .T. ) ;
#9351=CARTESIAN_POINT ( 'NONE',  ( 1.035533905932739085, -2.500000000000000000, -2.049999999999999822 ) ) ;
#9361=CARTESIAN_POINT ( 'NONE',  ( -1.461580736456472795, 1.461580736456472795, -2.049999998907525711 ) ) ;
#9364=AXIS2_PLACEMENT_3D ( 'NONE', #12737, #14012, #15138 ) ;
#9370=CARTESIAN_POINT ( 'NONE',  ( -2.066987299999999639, 0.000000000000000000, 2.250000001092474999 ) ) ;
#9390=CARTESIAN_POINT ( 'NONE',  ( -2.500000000000000000, -1.035533905932739307, -1.349999997815050090 ) ) ;
#9391=FACE_OUTER_BOUND ( 'NONE', #14905, .T. ) ;
#9393=CARTESIAN_POINT ( 'NONE',  ( -1.035533905932737753, 2.500000000000000444, 0.7499999999999998890 ) ) ;
#9394=CARTESIAN_POINT ( 'NONE',  ( -2.066987299999999195, -0.8561741729129466183, -2.499999998907525001 ) ) ;
#9404=CARTESIAN_POINT ( 'NONE',  ( 2.066987299999999639, 2.531329380823229670E-16, 1.650000001092474911 ) ) ;
#9409=CARTESIAN_POINT ( 'NONE',  ( 4.592425496802573972E-16, -2.500000000000000000, 0.3069999999781504174 ) ) ;
#9414=CARTESIAN_POINT ( 'NONE',  ( 1.461580736456473018, -1.461580736456472573, -0.04999999890752549608 ) ) ;
#9427=DIRECTION ( 'NONE',  ( 0.000000000000000000, 0.000000000000000000, -1.000000000000000000 ) ) ;
#9432=CARTESIAN_POINT ( 'NONE',  ( 4.592425496802573972E-16, -2.500000000000000000, 0.2999999999999999334 ) ) ;
#9434=( NAMED_UNIT ( * ) PLANE_ANGLE_UNIT ( ) SI_UNIT ( $, .RADIAN. ) );
#9451=CARTESIAN_POINT ( 'NONE',  ( 2.500000000000000000, 3.061616997868383141E-16, -0.1999999978150501789 ) ) ;
#9456=CARTESIAN_POINT ( 'NONE',  ( -0.8561741729129458411, -2.066987299999999195, 1.092474635061568626E-09 ) ) ;
#9466=CIRCLE ( 'NONE', #10986, 1.500000000000000000 ) ;
#9471=CARTESIAN_POINT ( 'NONE',  ( -2.500000000000000000, -1.035533905932739307, 1.050000002184949821 ) ) ;
#9478=ORIENTED_EDGE ( 'NONE', *, *, #11959, .F. ) ;
#9486=CARTESIAN_POINT ( 'NONE',  ( -1.530808498934191571E-16, 2.500000000000000000, -3.199999997815050623 ) ) ;
#9490=CARTESIAN_POINT ( 'NONE',  ( -1.767766952966369098, 1.767766952966369098, -1.593000000021849827 ) ) ;
#9493=CARTESIAN_POINT ( 'NONE',  ( 2.066987299999999639, 2.531329380823229670E-16, 0.8500000010924746441 ) ) ;
#9512=CARTESIAN_POINT ( 'NONE',  ( -2.500000000000000000, -1.035533905932739307, -2.250000000000000444 ) ) ;
#9527=ORIENTED_EDGE ( 'NONE', *, *, #1853, .F. ) ;
#9530=CARTESIAN_POINT ( 'NONE',  ( 1.461580736456472573, 1.461580736456472795, 1.950000001092474955 ) ) ;
#9537=CARTESIAN_POINT ( 'NONE',  ( 2.066987299999999639, 2.531329380823229670E-16, 1.850000001092474866 ) ) ;
#9553=CARTESIAN_POINT ( 'NONE',  ( 2.500000000000000000, 3.061616997868383141E-16, 0.6000000021849497545 ) ) ;
#9564=CARTESIAN_POINT ( 'NONE',  ( -2.500000000000000444, 1.035533905932737753, -3.049999997815050268 ) ) ;
#9566=CARTESIAN_POINT ( 'NONE',  ( -2.500000000000000444, 1.035533905932737753, 0.05000000000000013461 ) ) ;
#9568=CARTESIAN_POINT ( 'NONE',  ( 2.500000000000000444, -1.035533905932737309, -0.3430000000218496048 ) ) ;
#9571=CARTESIAN_POINT ( 'NONE',  ( -1.461580736456472795, 1.461580736456472795, -2.849999998907525089 ) ) ;
#9579=ORIENTED_EDGE ( 'NONE', *, *, #10572, .F. ) ;
#9598=ADVANCED_FACE ( 'NONE', ( #11756 ), #15508, .F. ) ;
#9607=VERTEX_POINT ( 'NONE', #1018 ) ;
#9608=DIRECTION ( 'NONE',  ( 0.8660254037844400399, 0.000000000000000000, 0.4999999999999975020 ) ) ;
#9613=CARTESIAN_POINT ( 'NONE',  ( -0.8561741729129455081, 2.066987299999999639, 1.300000001092474822 ) ) ;
#9622=CARTESIAN_POINT ( 'NONE',  ( 3.796994071234844259E-16, -2.066987299999999639, 0.05000000109247476621 ) ) ;
#9626=VECTOR ( 'NONE', #1861, 1000.000000000000000 ) ;
#9630=( NAMED_UNIT ( * ) PLANE_ANGLE_UNIT ( ) SI_UNIT ( $, .RADIAN. ) );
#9635=DIRECTION ( 'NONE',  ( -0.8660254037844387076, -0.4999999999999998890, 0.000000000000000000 ) ) ;
#9636=CARTESIAN_POINT ( 'NONE',  ( -3.000000000000000000, 1.732050807568877415, -5.500000000000000000 ) ) ;
#9639=CARTESIAN_POINT ( 'NONE',  ( 2.500000000000000444, 1.035533905932737975, 0.5499999999999999334 ) ) ;
#9650=CARTESIAN_POINT ( 'NONE',  ( -2.066987299999999639, 0.000000000000000000, 2.050000001092474822 ) ) ;
#9654=CARTESIAN_POINT ( 'NONE',  ( -1.767766952966368432, -1.767766952966369320, 1.006999999978150484 ) ) ;
#9658=CARTESIAN_POINT ( 'NONE',  ( 2.066987299999999639, 2.531329380823229670E-16, -2.349999998907525534 ) ) ;
#9662=ORIENTED_EDGE ( 'NONE', *, *, #7211, .T. ) ;
#9671=( BOUNDED_CURVE ( )  B_SPLINE_CURVE ( 2, ( #13035, #5889, #3407, #12874, #8038, #15278, #9309, #10655, #15435 ),
 .UNSPECIFIED., .F., .F. ) 
 B_SPLINE_CURVE_WITH_KNOTS ( ( 3, 2, 2, 2, 3 ),
 ( 0.2857142857142856984, 0.3035714285714285476, 0.3214285714285714524, 0.3392857142857143016, 0.3571428571428571508 ),
 .UNSPECIFIED. ) 
 CURVE ( )  GEOMETRIC_REPRESENTATION_ITEM ( )  RATIONAL_B_SPLINE_CURVE ( ( 1.000000000000000000, 0.9238795325112867385, 1.000000000000000000, 0.9238795325112867385, 1.000000000000000000, 0.9238795325112867385, 1.000000000000000000, 0.9238795325112867385, 1.000000000000000000 ) ) 
 REPRESENTATION_ITEM ( '' )  );
#9676=CARTESIAN_POINT ( 'NONE',  ( 2.500000000000000000, 3.061616997868383141E-16, -0.9999999978150501123 ) ) ;
#9695=CARTESIAN_POINT ( 'NONE',  ( 2.066987300000000083, -0.8561741729129449530, 1.000000001092474777 ) ) ;
#9702=CARTESIAN_POINT ( 'NONE',  ( -1.461580736456472351, -1.461580736456473018, 0.7500000010924748883 ) ) ;
#9719=CARTESIAN_POINT ( 'NONE',  ( -2.500000000000000444, 1.035533905932737753, -2.249999997815050445 ) ) ;
#9722=EDGE_CURVE ( 'NONE', #15372, #26, #6422, .T. ) ;
#9729=VECTOR ( 'NONE', #7186, 1000.000000000000114 ) ;
#9732=CARTESIAN_POINT ( 'NONE',  ( 2.066987299999999639, 0.8561741729129456191, 1.700000001092474733 ) ) ;
#9737=CARTESIAN_POINT ( 'NONE',  ( 0.9662756667218489470, 2.500000000000000000, -2.539655916413669168 ) ) ;
#9740=CARTESIAN_POINT ( 'NONE',  ( 0.8561741729129463963, -2.066987299999999195, -2.499999998907525445 ) ) ;
#9748=ORIENTED_EDGE ( 'NONE', *, *, #9844, .T. ) ;
#9761=EDGE_CURVE ( 'NONE', #546, #10381, #6962, .T. ) ;
#9770=CARTESIAN_POINT ( 'NONE',  ( 1.035533905932737531, 2.500000000000000444, -0.9500000000000003997 ) ) ;
#9774=CARTESIAN_POINT ( 'NONE',  ( 1.461580736456473018, -1.461580736456472573, 0.1500000010924746052 ) ) ;
#9778=CARTESIAN_POINT ( 'NONE',  ( 2.500000000000000444, -1.035533905932737309, -1.849999997815050090 ) ) ;
#9780=CARTESIAN_POINT ( 'NONE',  ( 2.066987299999999639, 0.8561741729129456191, 1.900000001092474911 ) ) ;
#9785=CARTESIAN_POINT ( 'NONE',  ( -1.464522546803547017E-16, 2.391746824999999799, -2.562499999726881139 ) ) ;
#9787=EDGE_LOOP ( 'NONE', ( #2962, #10690, #7835, #11866, #14865, #1603 ) ) ;
#9788=PRESENTATION_STYLE_ASSIGNMENT (( #8521 ) ) ;
#9793=CARTESIAN_POINT ( 'NONE',  ( -1.767766952966368432, -1.767766952966369320, -2.899999997815050357 ) ) ;
#9799=EDGE_CURVE ( 'NONE', #4492, #15063, #914, .T. ) ;
#9805=VERTEX_POINT ( 'NONE', #12152 ) ;
#9806=CARTESIAN_POINT ( 'NONE',  ( -2.066987299999999639, 0.8561741729129452860, -1.199999998907525622 ) ) ;
#9809=CARTESIAN_POINT ( 'NONE',  ( -1.530808498934191571E-16, 2.500000000000000000, -0.1000000000000002554 ) ) ;
#9811=CARTESIAN_POINT ( 'NONE',  ( -1.035533905932738197, -2.500000000000000000, -2.143000000021849871 ) ) ;
#9816=CARTESIAN_POINT ( 'NONE',  ( -2.066987299999999639, 0.8561741729129452860, 1.400000001092474911 ) ) ;
#9828=CARTESIAN_POINT ( 'NONE',  ( -1.265664690411614835E-16, 2.066987299999999639, -2.949999998907525178 ) ) ;
#9833=ADVANCED_FACE ( 'NONE', ( #5002 ), #11993, .F. ) ;
#9844=EDGE_CURVE ( 'NONE', #9302, #4950, #15566, .T. ) ;
#9846=CARTESIAN_POINT ( 'NONE',  ( -2.066987299999999639, 0.000000000000000000, 1.450000001092474955 ) ) ;
#9851=CARTESIAN_POINT ( 'NONE',  ( -2.500000000000000000, -1.035533905932739307, -2.149999997815051245 ) ) ;
#9854=CARTESIAN_POINT ( 'NONE',  ( -1.461580736456472351, -1.461580736456473018, -1.649999998907525356 ) ) ;
#9857=CARTESIAN_POINT ( 'NONE',  ( -1.461580736456472795, 1.461580736456472795, 1.150000001092474688 ) ) ;
#9863=( NAMED_UNIT ( * ) SI_UNIT ( $, .STERADIAN. ) SOLID_ANGLE_UNIT ( ) );
#9881=ORIENTED_EDGE ( 'NONE', *, *, #12792, .F. ) ;
#9883=CARTESIAN_POINT ( 'NONE',  ( -0.8561741729129458411, -2.066987299999999195, -0.1999999989075254836 ) ) ;
#9888=CARTESIAN_POINT ( 'NONE',  ( -2.500000000000000000, -1.035533905932739307, 1.750000000000000222 ) ) ;
#9892=CARTESIAN_POINT ( 'NONE',  ( -2.066987299999999639, 0.8561741729129452860, -1.999999998907524779 ) ) ;
#9915=( GEOMETRIC_REPRESENTATION_CONTEXT ( 3 ) GLOBAL_UNCERTAINTY_ASSIGNED_CONTEXT ( ( #11660 ) ) GLOBAL_UNIT_ASSIGNED_CONTEXT ( ( #1945, #9434, #7131 ) ) REPRESENTATION_CONTEXT ( 'NONE', 'WORKASPACE' ) );
#9923=CARTESIAN_POINT ( 'NONE',  ( 2.500000000000000444, 1.035533905932737975, 2.149999999999999911 ) ) ;
#9927=CARTESIAN_POINT ( 'NONE',  ( -1.500000000000000000, 0.000000000000000000, 2.500000000000000000 ) ) ;
#9929=CARTESIAN_POINT ( 'NONE',  ( 2.500000000000000000, 3.061616997868383141E-16, -1.799999997815050490 ) ) ;
#9931=CARTESIAN_POINT ( 'NONE',  ( -2.066987299999999639, 0.000000000000000000, -1.749999998907525223 ) ) ;
#9933=CARTESIAN_POINT ( 'NONE',  ( -0.8561741729129458411, -2.066987299999999195, 1.400000001092474911 ) ) ;
#9945=CARTESIAN_POINT ( 'NONE',  ( -1.767766952966368432, -1.767766952966369320, 0.2000000000000000944 ) ) ;
#9946=CARTESIAN_POINT ( 'NONE',  ( 1.035533905932739085, -2.500000000000000000, -2.749999997815050445 ) ) ;
#9961=CARTESIAN_POINT ( 'NONE',  ( 1.461580736456472573, 1.461580736456472795, 0.1500000010924747995 ) ) ;
#9965=CARTESIAN_POINT ( 'NONE',  ( 4.592425496802573972E-16, -2.500000000000000000, 1.899999999999999911 ) ) ;
#9970=CARTESIAN_POINT ( 'NONE',  ( 1.461580736456472573, 1.461580736456472795, -0.4499999989075252338 ) ) ;
#9995=ORIENTED_EDGE ( 'NONE', *, *, #4632, .T. ) ;
#10004=CARTESIAN_POINT ( 'NONE',  ( -1.035533905932737753, 2.500000000000000444, 1.550000000000000044 ) ) ;
#10011=CARTESIAN_POINT ( 'NONE',  ( 0.8561741729129465073, -2.066987299999999195, -1.499999998907525445 ) ) ;
#10013=CARTESIAN_POINT ( 'NONE',  ( -2.066987299999999195, -0.8561741729129467293, 1.300000001092474600 ) ) ;
#10017=EDGE_LOOP ( 'NONE', ( #5882, #9023, #1273 ) ) ;
#10028=EDGE_CURVE ( 'NONE', #12110, #11794, #14536, .T. ) ;
#10030=ORIENTED_EDGE ( 'NONE', *, *, #9761, .T. ) ;
#10039=CARTESIAN_POINT ( 'NONE',  ( 3.796994071234844259E-16, -2.066987299999999639, -0.9499999989075252893 ) ) ;
#10043=CARTESIAN_POINT ( 'NONE',  ( 1.767766952966368654, 1.767766952966369098, 2.200000000000000178 ) ) ;
#10048=CARTESIAN_POINT ( 'NONE',  ( 2.066987300000000083, -0.8561741729129449530, -0.5999999989075250895 ) ) ;
#10071=ORIENTED_EDGE ( 'NONE', *, *, #12700, .T. ) ;
#10078=CARTESIAN_POINT ( 'NONE',  ( 2.500000000000000444, -1.035533905932737309, 2.049999999999999822 ) ) ;
#10087=CARTESIAN_POINT ( 'NONE',  ( -2.500000000000000444, 1.035533905932737753, -3.049999997815050268 ) ) ;
#10097=EDGE_CURVE ( 'NONE', #338, #10381, #7027, .T. ) ;
#10116=CARTESIAN_POINT ( 'NONE',  ( 2.066987299999999639, 2.531329380823229670E-16, -0.7499999989075251117 ) ) ;
#10121=CARTESIAN_POINT ( 'NONE',  ( -1.530808498934191571E-16, 2.500000000000000000, 1.600000002184949865 ) ) ;
#10122=CARTESIAN_POINT ( 'NONE',  ( -1.767766952966368432, -1.767766952966369320, -1.400000000000000133 ) ) ;
#10123=AXIS2_PLACEMENT_3D ( 'NONE', #2464, #1344, #14643 ) ;
#10125=CARTESIAN_POINT ( 'NONE',  ( 2.500000000000000000, 3.061616997868383141E-16, -0.9999999978150501123 ) ) ;
#10126=CARTESIAN_POINT ( 'NONE',  ( 3.796994071234844259E-16, -2.066987299999999639, -1.549999998907525045 ) ) ;
#10129=DIRECTION ( 'NONE',  ( -1.000000000000000000, 0.000000000000000000, 0.000000000000000000 ) ) ;
#10140=CARTESIAN_POINT ( 'NONE',  ( 2.500000000000000000, 3.061616997868383141E-16, -1.900000000000000133 ) ) ;
#10151=ORIENTED_EDGE ( 'NONE', *, *, #6320, .T. ) ;
#10159=CARTESIAN_POINT ( 'NONE',  ( -2.500000000000000000, 0.000000000000000000, 2.500000000000000000 ) ) ;
#10164=CARTESIAN_POINT ( 'NONE',  ( -2.066987299999999639, 0.000000000000000000, -2.549999998907525711 ) ) ;
#10166=CARTESIAN_POINT ( 'NONE',  ( -0.8561741729129455081, 2.066987299999999639, 1.100000001092475088 ) ) ;
#10196=CARTESIAN_POINT ( 'NONE',  ( 1.035533905932737531, 2.500000000000000444, -1.750000000000000222 ) ) ;
#10198=CARTESIAN_POINT ( 'NONE',  ( 1.767766952966369320, -1.767766952966368654, -1.200000000000000178 ) ) ;
#10203=CARTESIAN_POINT ( 'NONE',  ( -0.8561741729129458411, -2.066987299999999195, 1.092474635061568626E-09 ) ) ;
#10217=CARTESIAN_POINT ( 'NONE',  ( -1.767766952966369098, 1.767766952966369098, 2.406999999978150395 ) ) ;
#10225=VERTEX_POINT ( 'NONE', #6286 ) ;
#10226=CARTESIAN_POINT ( 'NONE',  ( -1.698715844156870602, 1.839699740483268675, -2.499564404588821898 ) ) ;
#10237=CARTESIAN_POINT ( 'NONE',  ( 2.066987300000000083, -0.8561741729129449530, -1.399999998907525134 ) ) ;
#10246=CARTESIAN_POINT ( 'NONE',  ( 0.8561741729129465073, -2.066987299999999195, -2.499999998907525445 ) ) ;
#10257=CARTESIAN_POINT ( 'NONE',  ( -1.265664690411614835E-16, 2.066987299999999639, -2.949999998907525178 ) ) ;
#10261=ORIENTED_EDGE ( 'NONE', *, *, #11959, .T. ) ;
#10273=CARTESIAN_POINT ( 'NONE',  ( 2.500000000000000444, 1.035533905932737975, -1.050000000000000044 ) ) ;
#10274=CARTESIAN_POINT ( 'NONE',  ( 1.767766952966368654, 1.767766952966369098, 2.200000000000000178 ) ) ;
#10278=CARTESIAN_POINT ( 'NONE',  ( 2.066987299999999639, 0.8561741729129456191, -1.299999998907525267 ) ) ;
#10287=ORIENTED_EDGE ( 'NONE', *, *, #15038, .F. ) ;
#10289=CARTESIAN_POINT ( 'NONE',  ( -1.530808498934191571E-16, 2.500000000000000000, -0.7999999978150507118 ) ) ;
#10303=CARTESIAN_POINT ( 'NONE',  ( -1.983218494070152493, 1.528667308324898944, -2.500812883383392915 ) ) ;
#10308=CARTESIAN_POINT ( 'NONE',  ( 0.000000000000000000, 0.000000000000000000, 2.500000000000000000 ) ) ;
#10309=DIRECTION ( 'NONE',  ( 0.000000000000000000, 0.000000000000000000, -1.000000000000000000 ) ) ;
#10311=CARTESIAN_POINT ( 'NONE',  ( -1.035533905932738197, -2.500000000000000000, 1.850000000000000311 ) ) ;
#10312=CARTESIAN_POINT ( 'NONE',  ( -2.500000000000000444, 1.035533905932737753, -0.7500000000000004441 ) ) ;
#10320=CARTESIAN_POINT ( 'NONE',  ( 1.461580736456473018, -1.461580736456472573, -1.649999998907525356 ) ) ;
#10344=DIRECTION ( 'NONE',  ( 1.251928832280965695E-16, 1.000000000000000000, 0.000000000000000000 ) ) ;
#10349=CARTESIAN_POINT ( 'NONE',  ( -1.035533905932737753, 2.500000000000000444, 1.650000002184949910 ) ) ;
#10350=CARTESIAN_POINT ( 'NONE',  ( 4.592425496802573972E-16, -2.500000000000000000, -1.300000000000000044 ) ) ;
#10353=CARTESIAN_POINT ( 'NONE',  ( -1.084202172485504434E-16, 3.464101615137754830, -5.500000000000000000 ) ) ;
#10366=CARTESIAN_POINT ( 'NONE',  ( 2.500000000000000444, -1.035533905932737309, 0.5500000021849495990 ) ) ;
#10370=CARTESIAN_POINT ( 'NONE',  ( 2.500000000000000000, 3.061616997868383141E-16, 2.106999999978150129 ) ) ;
#10374=CARTESIAN_POINT ( 'NONE',  ( 2.066987299999999639, 0.8561741729129456191, 1.700000001092474733 ) ) ;
#10380=CARTESIAN_POINT ( 'NONE',  ( -2.515015366234329530, -0.07938793225241053131, -2.500633784899425560 ) ) ;
#10381=VERTEX_POINT ( 'NONE', #12840 ) ;
#10393=CARTESIAN_POINT ( 'NONE',  ( -2.500000000000000000, -1.035533905932739307, -1.450000000000000400 ) ) ;
#10400=CARTESIAN_POINT ( 'NONE',  ( 2.066987299999999639, 2.531329380823229670E-16, -0.7499999989075251117 ) ) ;
#10406=EDGE_CURVE ( 'NONE', #15622, #4492, #2553, .T. ) ;
#10417=CARTESIAN_POINT ( 'NONE',  ( 2.500000000000000000, 3.061616997868383141E-16, 1.400000002184949910 ) ) ;
#10418=ORIENTED_EDGE ( 'NONE', *, *, #5519, .T. ) ;
#10431=CARTESIAN_POINT ( 'NONE',  ( 2.500000000000000444, -1.035533905932737309, -1.949999999999999956 ) ) ;
#10444=CARTESIAN_POINT ( 'NONE',  ( 2.500000000000000444, -1.035533905932737309, -0.2499999978150505286 ) ) ;
#10448=CARTESIAN_POINT ( 'NONE',  ( -1.035533905932737753, 2.500000000000000444, 1.556999999978150750 ) ) ;
#10452=CARTESIAN_POINT ( 'NONE',  ( -1.461580736456472351, -1.461580736456473018, 0.5500000010924748217 ) ) ;
#10458=CARTESIAN_POINT ( 'NONE',  ( 4.592425496802573972E-16, -2.500000000000000000, 0.4000000021849499099 ) ) ;
#10467=CARTESIAN_POINT ( 'NONE',  ( 4.592425496802573972E-16, -2.500000000000000000, -0.5000000000000000000 ) ) ;
#10477=CARTESIAN_POINT ( 'NONE',  ( 0.8561741729129452860, 2.066987299999999639, -0.5999999989075253115 ) ) ;
#10485=ORIENTED_EDGE ( 'NONE', *, *, #10028, .T. ) ;
#10489=CARTESIAN_POINT ( 'NONE',  ( 1.767766952966369320, -1.767766952966368654, -0.2999999978150504343 ) ) ;
#10494=CARTESIAN_POINT ( 'NONE',  ( -2.500000000000000000, 0.000000000000000000, 2.150000001092474911 ) ) ;
#10501=ADVANCED_BREP_SHAPE_REPRESENTATION ( '', ( #5230, #14201 ), #6617 ) ;
#10507=CARTESIAN_POINT ( 'NONE',  ( 1.035533905932739085, -2.500000000000000000, -1.149999997815050135 ) ) ;
#10522=CARTESIAN_POINT ( 'NONE',  ( -1.767766952966369098, 1.767766952966369098, 0.9000000021849495768 ) ) ;
#10526=CARTESIAN_POINT ( 'NONE',  ( 2.500000000000000000, 3.061616997868383141E-16, -1.893000000021849649 ) ) ;
#10529=CARTESIAN_POINT ( 'NONE',  ( 2.066987299999999639, 2.531329380823229670E-16, 1.650000001092474911 ) ) ;
#10534=CARTESIAN_POINT ( 'NONE',  ( 1.264010580706230957, -2.175748604140837816, -2.499149807554369218 ) ) ;
#10543=CARTESIAN_POINT ( 'NONE',  ( -1.767766952966369098, 1.767766952966369098, 0.7999999999999999334 ) ) ;
#10546=CYLINDRICAL_SURFACE ( 'NONE', #9022, 2.500000000000000000 ) ;
#10572=EDGE_CURVE ( 'NONE', #5999, #9607, #4172, .T. ) ;
#10580=CARTESIAN_POINT ( 'NONE',  ( -1.530808498934191571E-16, 2.500000000000000000, -0.7999999978150504898 ) ) ;
#10584=CARTESIAN_POINT ( 'NONE',  ( 0.8561741729129463963, -2.066987299999999195, -2.299999998907525267 ) ) ;
#10595=CARTESIAN_POINT ( 'NONE',  ( 4.592425496802573972E-16, -2.500000000000000000, -1.199999997815050401 ) ) ;
#10600=CARTESIAN_POINT ( 'NONE',  ( 2.500000000000000444, 1.035533905932737975, 0.5569999999781504174 ) ) ;
#10603=CARTESIAN_POINT ( 'NONE',  ( -2.066987299999999639, 0.8561741729129452860, 0.4000000010924749105 ) ) ;
#10621=CARTESIAN_POINT ( 'NONE',  ( -2.500000000000000000, 0.000000000000000000, -1.399999997815050357 ) ) ;
#10622=CARTESIAN_POINT ( 'NONE',  ( -2.500000000000000000, 0.000000000000000000, 0.9000000000000000222 ) ) ;
#10634=DIRECTION ( 'NONE',  ( 0.000000000000000000, 0.000000000000000000, -1.000000000000000000 ) ) ;
#10638=CARTESIAN_POINT ( 'NONE',  ( -2.066987299999999639, 0.8561741729129452860, 2.200000001092475177 ) ) ;
#10640=CARTESIAN_POINT ( 'NONE',  ( 1.035533905932739085, -2.500000000000000000, -0.3499999978150501456 ) ) ;
#10645=CARTESIAN_POINT ( 'NONE',  ( 0.8561741729129465073, -2.066987299999999195, 1.700000001092474733 ) ) ;
#10655=CARTESIAN_POINT ( 'NONE',  ( 2.500000000000000444, 1.035533905932737975, -0.1499999978150502455 ) ) ;
#10659=CARTESIAN_POINT ( 'NONE',  ( 4.592425496802573972E-16, -2.500000000000000000, -0.3999999978150502455 ) ) ;
#10663=CARTESIAN_POINT ( 'NONE',  ( 2.500000000000000000, 3.061616997868383141E-16, 2.500000000000000000 ) ) ;
#10669=ORIENTED_EDGE ( 'NONE', *, *, #14948, .T. ) ;
#10670=ORIENTED_EDGE ( 'NONE', *, *, #553, .T. ) ;
#10675=CARTESIAN_POINT ( 'NONE',  ( -1.461580736456472351, -1.461580736456473018, 1.350000001092474644 ) ) ;
#10679=CARTESIAN_POINT ( 'NONE',  ( -2.500000000000000000, -1.035533905932739307, -1.443000000021849694 ) ) ;
#10682=CARTESIAN_POINT ( 'NONE',  ( -1.265664690411614835E-16, 2.066987299999999639, -0.5499999989075254891 ) ) ;
#10690=ORIENTED_EDGE ( 'NONE', *, *, #2387, .F. ) ;
#10696=FACE_OUTER_BOUND ( 'NONE', #5101, .T. ) ;
#10713=CYLINDRICAL_SURFACE ( 'NONE', #11318, 2.500000000000000000 ) ;
#10714=ORIENTED_EDGE ( 'NONE', *, *, #10406, .F. ) ;
#10719=CARTESIAN_POINT ( 'NONE',  ( -1.461580736456472351, -1.461580736456473018, 0.7500000010924748883 ) ) ;
#10726=CARTESIAN_POINT ( 'NONE',  ( 1.461580736456472573, 1.461580736456472795, -0.4499999989075252338 ) ) ;
#10740=CARTESIAN_POINT ( 'NONE',  ( 2.500000000000000444, 1.035533905932737975, -1.749999997815050667 ) ) ;
#10741=DIRECTION ( 'NONE',  ( -1.000000000000000000, 0.000000000000000000, 0.000000000000000000 ) ) ;
#10753=CARTESIAN_POINT ( 'NONE',  ( 2.500000000000000444, 1.035533905932737975, -1.749999997815050889 ) ) ;
#10756=CARTESIAN_POINT ( 'NONE',  ( 2.999999999999999556, -1.732050807568877859, -5.500000000000000000 ) ) ;
#10759=CARTESIAN_POINT ( 'NONE',  ( 4.592425496802573972E-16, -2.500000000000000000, -1.293000000021849338 ) ) ;
#10763=CARTESIAN_POINT ( 'NONE',  ( -1.461580736456472351, -1.461580736456473018, -1.049999998907525489 ) ) ;
#10767=ORIENTED_EDGE ( 'NONE', *, *, #3829, .T. ) ;
#10791=LINE ( 'NONE', #12657, #12414 ) ;
#10795=CARTESIAN_POINT ( 'NONE',  ( 3.796994071234844259E-16, -2.066987299999999639, -0.7499999989075251117 ) ) ;
#10797=ADVANCED_FACE ( 'NONE', ( #11402 ), #5807, .T. ) ;
#10803=CARTESIAN_POINT ( 'NONE',  ( -0.8561741729129455081, 2.066987299999999639, 2.100000001092475088 ) ) ;
#10804=CARTESIAN_POINT ( 'NONE',  ( -3.000000000000000000, 1.732050807568877415, -5.500000000000000000 ) ) ;
#10821=CARTESIAN_POINT ( 'NONE',  ( -2.500000000000000444, 1.035533905932737753, 0.8500000000000001998 ) ) ;
#10824=VERTEX_POINT ( 'NONE', #9636 ) ;
#10830=CARTESIAN_POINT ( 'NONE',  ( -2.500000000000000000, 0.000000000000000000, -2.999999997815050889 ) ) ;
#10834=CARTESIAN_POINT ( 'NONE',  ( -1.530808498934191571E-16, 2.500000000000000000, 0.7069999999781503286 ) ) ;
#10837=CARTESIAN_POINT ( 'NONE',  ( 2.066987300000000083, -0.8561741729129449530, -2.399999998907525356 ) ) ;
#10842=EDGE_LOOP ( 'NONE', ( #4552, #1387, #1970, #14563 ) ) ;
#10844=VERTEX_POINT ( 'NONE', #2381 ) ;
#10852=DIRECTION ( 'NONE',  ( -1.000000000000000000, 0.000000000000000000, 0.000000000000000000 ) ) ;
#10875=VECTOR ( 'NONE', #3362, 1000.000000000000000 ) ;
#10876=CARTESIAN_POINT ( 'NONE',  ( -2.066987299999999639, 0.000000000000000000, 2.150000001092474911 ) ) ;
#10878=CARTESIAN_POINT ( 'NONE',  ( -2.066987299999999639, 0.000000000000000000, -0.9499999989075252893 ) ) ;
#10885=CARTESIAN_POINT ( 'NONE',  ( -0.8561741729129455081, 2.066987299999999639, -0.2999999989075252671 ) ) ;
#10887=CARTESIAN_POINT ( 'NONE',  ( 1.035533905932737531, 2.500000000000000444, 1.450000000000000400 ) ) ;
#10901=CARTESIAN_POINT ( 'NONE',  ( -2.066987299999999639, 0.8561741729129452860, -0.9999999989075254447 ) ) ;
#10904=CARTESIAN_POINT ( 'NONE',  ( -2.283493650000000041, 0.000000000000000000, 2.375000000546237278 ) ) ;
#10914=EDGE_CURVE ( 'NONE', #5531, #6066, #13422, .T. ) ;
#10915=CARTESIAN_POINT ( 'NONE',  ( -2.066987299999999639, 0.000000000000000000, 1.250000001092474777 ) ) ;
#10916=DIRECTION ( 'NONE',  ( -0.5000000000000000000, -0.8660254037844387076, 0.000000000000000000 ) ) ;
#10919=CARTESIAN_POINT ( 'NONE',  ( -2.500000000000000000, -1.035533905932739307, 0.1499999999999999667 ) ) ;
#10921=CARTESIAN_POINT ( 'NONE',  ( -1.461580736456472795, 1.461580736456472795, 1.350000001092474644 ) ) ;
#10927=ORIENTED_EDGE ( 'NONE', *, *, #5703, .T. ) ;
#10946=CARTESIAN_POINT ( 'NONE',  ( 0.000000000000000000, 0.000000000000000000, 2.500000000000000000 ) ) ;
#10953=CARTESIAN_POINT ( 'NONE',  ( -1.461580736456472351, -1.461580736456473018, -0.8499999989075254225 ) ) ;
#10961=CARTESIAN_POINT ( 'NONE',  ( 2.066987299999999639, 2.531329380823229670E-16, 0.2500000010924748328 ) ) ;
#10970=SURFACE_SIDE_STYLE ('',( #12159 ) ) ;
#10986=AXIS2_PLACEMENT_3D ( 'NONE', #8580, #12214, #13253 ) ;
#10991=CARTESIAN_POINT ( 'NONE',  ( 1.035533905932739085, -2.500000000000000000, -1.949999997815050401 ) ) ;
#10995=CARTESIAN_POINT ( 'NONE',  ( -1.767766952966368432, -1.767766952966369320, 1.000000000000000000 ) ) ;
#10998=CARTESIAN_POINT ( 'NONE',  ( 2.066987299999999639, 0.8561741729129456191, 1.900000001092474688 ) ) ;
#11009=LINE ( 'NONE', #8401, #6082 ) ;
#11031=CARTESIAN_POINT ( 'NONE',  ( 2.066987299999999639, 2.531329380823229670E-16, 1.050000001092474822 ) ) ;
#11039=CARTESIAN_POINT ( 'NONE',  ( 2.500000000000000444, 1.035533905932737975, 1.350000000000000089 ) ) ;
#11040=ORIENTED_EDGE ( 'NONE', *, *, #3699, .T. ) ;
#11041=CARTESIAN_POINT ( 'NONE',  ( 1.461580736456473018, -1.461580736456472573, 0.7500000010924746663 ) ) ;
#11052=CARTESIAN_POINT ( 'NONE',  ( -2.500000000000000000, -1.035533905932739307, 0.1499999999999999944 ) ) ;
#11053=CARTESIAN_POINT ( 'NONE',  ( -2.500000000000000000, -1.035533905932739307, -2.149999997815051245 ) ) ;
#11056=CARTESIAN_POINT ( 'NONE',  ( -1.767766952966369098, 1.767766952966369098, -2.299999997815050712 ) ) ;
#11066=CARTESIAN_POINT ( 'NONE',  ( -0.8561741729129455081, 2.066987299999999639, 0.3000000010924747662 ) ) ;
#11067=EDGE_CURVE ( 'NONE', #202, #546, #8663, .T. ) ;
#11071=CARTESIAN_POINT ( 'NONE',  ( -1.530808498934191571E-16, 2.500000000000000000, -2.493000000021849516 ) ) ;
#11075=CARTESIAN_POINT ( 'NONE',  ( 3.796994071234844259E-16, -2.066987299999999639, -2.549999998907525267 ) ) ;
#11081=ORIENTED_EDGE ( 'NONE', *, *, #12512, .T. ) ;
#11093=CARTESIAN_POINT ( 'NONE',  ( -1.530808498934191571E-16, 2.500000000000000000, 2.299999999999999822 ) ) ;
#11105=CARTESIAN_POINT ( 'NONE',  ( 2.999999999999999556, -1.732050807568877859, -2.500000000000000000 ) ) ;
#11106=EDGE_CURVE ( 'NONE', #1290, #13408, #1321, .T. ) ;
#11108=CARTESIAN_POINT ( 'NONE',  ( -1.461580736456472795, 1.461580736456472795, -2.649999998907524912 ) ) ;
#11113=DIRECTION ( 'NONE',  ( 0.000000000000000000, 0.000000000000000000, -1.000000000000000000 ) ) ;
#11116=DIRECTION ( 'NONE',  ( 0.000000000000000000, 0.000000000000000000, -1.000000000000000000 ) ) ;
#11119=CARTESIAN_POINT ( 'NONE',  ( -1.461580736456472795, 1.461580736456472795, 0.3500000010924746996 ) ) ;
#11132=CARTESIAN_POINT ( 'NONE',  ( -1.035533905932737753, 2.500000000000000444, -3.149999997815050801 ) ) ;
#11145=AXIS2_PLACEMENT_3D ( 'NONE', #7642, #3741, #4872 ) ;
#11146=CARTESIAN_POINT ( 'NONE',  ( 3.796994071234844259E-16, -2.066987299999999639, 0.6500000010924747995 ) ) ;
#11150=CARTESIAN_POINT ( 'NONE',  ( -1.767766952966368432, -1.767766952966369320, -2.193000000021849694 ) ) ;
#11154=CARTESIAN_POINT ( 'NONE',  ( 0.8561741729129463963, -2.066987299999999195, 0.1000000010924748939 ) ) ;
#11158=ORIENTED_EDGE ( 'NONE', *, *, #2387, .T. ) ;
#11159=EDGE_LOOP ( 'NONE', ( #11158, #922, #2945, #7240 ) ) ;
#11178=( GEOMETRIC_REPRESENTATION_CONTEXT ( 3 ) GLOBAL_UNCERTAINTY_ASSIGNED_CONTEXT ( ( #5851 ) ) GLOBAL_UNIT_ASSIGNED_CONTEXT ( ( #6210, #9630, #9863 ) ) REPRESENTATION_CONTEXT ( 'NONE', 'WORKASPACE' ) );
#11185=CARTESIAN_POINT ( 'NONE',  ( -2.500000000000000000, 0.000000000000000000, 2.500000000000000000 ) ) ;
#11187=CARTESIAN_POINT ( 'NONE',  ( 0.8561741729129451750, 2.066987299999999639, -1.999999998907525223 ) ) ;
#11203=CARTESIAN_POINT ( 'NONE',  ( -1.265664690411614835E-16, 2.066987299999999639, -2.749999998907525001 ) ) ;
#11223=CARTESIAN_POINT ( 'NONE',  ( -1.265664690411614835E-16, 2.066987299999999639, -0.5499999989075254891 ) ) ;
#11227=CARTESIAN_POINT ( 'NONE',  ( 2.500000000000000444, 1.035533905932737975, 1.350000000000000089 ) ) ;
#11231=CARTESIAN_POINT ( 'NONE',  ( -1.461580736456472795, 1.461580736456472795, -1.049999998907525045 ) ) ;
#11265=CARTESIAN_POINT ( 'NONE',  ( -1.035533905932738197, -2.500000000000000000, 1.050000000000000044 ) ) ;
#11275=CARTESIAN_POINT ( 'NONE',  ( -2.066987299999999639, 0.8561741729129455081, 2.000000001092474555 ) ) ;
#11302=CARTESIAN_POINT ( 'NONE',  ( -0.8561741729129458411, -2.066987299999999195, -1.799999998907525267 ) ) ;
#11306=CARTESIAN_POINT ( 'NONE',  ( -1.767766952966369098, 1.767766952966369098, -0.7999999999999999334 ) ) ;
#11310=CARTESIAN_POINT ( 'NONE',  ( 1.461580736456473018, -1.461580736456472573, -1.449999998907525178 ) ) ;
#11313=ORIENTED_EDGE ( 'NONE', *, *, #15384, .F. ) ;
#11318=AXIS2_PLACEMENT_3D ( 'NONE', #8174, #10634, #4432 ) ;
#11333=EDGE_CURVE ( 'NONE', #13466, #15372, #1425, .T. ) ;
#11342=CARTESIAN_POINT ( 'NONE',  ( -2.500000000000000444, 1.035533905932737753, 2.449999999999999734 ) ) ;
#11352=CARTESIAN_POINT ( 'NONE',  ( -1.461580736456472795, 1.461580736456472795, 1.950000001092474733 ) ) ;
#11377=CARTESIAN_POINT ( 'NONE',  ( 0.8561741729129451750, 2.066987299999999639, -0.5999999989075250895 ) ) ;
#11381=CARTESIAN_POINT ( 'NONE',  ( -2.500000000000000000, 0.000000000000000000, -2.300000000000000266 ) ) ;
#11386=CARTESIAN_POINT ( 'NONE',  ( -2.066987299999999639, 0.8561741729129452860, -0.1999999989075250117 ) ) ;
#11387=DIRECTION ( 'NONE',  ( 0.000000000000000000, 0.000000000000000000, -1.000000000000000000 ) ) ;
#11389=ADVANCED_FACE ( 'NONE', ( #5623 ), #10546, .T. ) ;
#11396=ORIENTED_EDGE ( 'NONE', *, *, #3699, .F. ) ;
#11402=FACE_OUTER_BOUND ( 'NONE', #7556, .T. ) ;
#11409=CARTESIAN_POINT ( 'NONE',  ( 1.915978517174143692, -1.631420465661153951, -2.500869043012635462 ) ) ;
#11413=CIRCLE ( 'NONE', #14732, 1.500000000000000000 ) ;
#11419=CARTESIAN_POINT ( 'NONE',  ( 1.461580736456472573, 1.461580736456472795, -2.049999998907525267 ) ) ;
#11428=CARTESIAN_POINT ( 'NONE',  ( 2.066987299999999639, 0.8561741729129456191, -2.299999998907525711 ) ) ;
#11454=CARTESIAN_POINT ( 'NONE',  ( -2.066987299999999639, 0.000000000000000000, -2.749999998907525445 ) ) ;
#11457=CARTESIAN_POINT ( 'NONE',  ( 2.500000000000000000, 3.061616997868383141E-16, -0.2999999999999999334 ) ) ;
#11463=CARTESIAN_POINT ( 'NONE',  ( -1.461580736456472795, 1.461580736456472795, -1.849999998907525534 ) ) ;
#11471=CARTESIAN_POINT ( 'NONE',  ( 1.035533905932739085, -2.500000000000000000, -0.3499999978150503677 ) ) ;
#11493=DIRECTION ( 'NONE',  ( 0.000000000000000000, 0.000000000000000000, -1.000000000000000000 ) ) ;
#11495=CARTESIAN_POINT ( 'NONE',  ( -1.035533905932738197, -2.500000000000000000, -0.5500000000000001554 ) ) ;
#11504=CARTESIAN_POINT ( 'NONE',  ( 1.461580736456472573, 1.461580736456472795, -1.449999998907525178 ) ) ;
#11513=DIRECTION ( 'NONE',  ( 0.000000000000000000, 0.000000000000000000, 1.000000000000000000 ) ) ;
#11530=CARTESIAN_POINT ( 'NONE',  ( -1.084202172485504434E-15, -3.464101615137755275, -5.500000000000000000 ) ) ;
#11532=CARTESIAN_POINT ( 'NONE',  ( -1.530808498934191571E-16, 2.500000000000000000, -1.700000000000000622 ) ) ;
#11540=ORIENTED_EDGE ( 'NONE', *, *, #7368, .T. ) ;
#11544=DIRECTION ( 'NONE',  ( -1.000000000000000000, 0.000000000000000000, 0.000000000000000000 ) ) ;
#11549=CARTESIAN_POINT ( 'NONE',  ( -1.767766952966368432, -1.767766952966369320, 0.3000000021849495990 ) ) ;
#11557=CARTESIAN_POINT ( 'NONE',  ( -2.500000000000000000, 0.000000000000000000, -0.7000000000000000666 ) ) ;
#11563=CARTESIAN_POINT ( 'NONE',  ( 0.02052235255247245385, -2.503876325069105402, -2.499973232076210472 ) ) ;
#11567=DIRECTION ( 'NONE',  ( 0.8660254037844385966, 0.4999999999999998890, 0.000000000000000000 ) ) ;
#11573=CARTESIAN_POINT ( 'NONE',  ( 1.035533905932739085, -2.500000000000000000, 0.3500000000000000333 ) ) ;
#11576=CARTESIAN_POINT ( 'NONE',  ( -2.500000000000000444, 1.035533905932737753, 1.750000002184949999 ) ) ;
#11582=CARTESIAN_POINT ( 'NONE',  ( 2.066987300000000083, -0.8561741729129450640, -2.399999998907525356 ) ) ;
#11589=CARTESIAN_POINT ( 'NONE',  ( -1.461580736456472795, 1.461580736456472795, 2.150000001092474911 ) ) ;
#11604=ORIENTED_EDGE ( 'NONE', *, *, #15038, .T. ) ;
#11609=LINE ( 'NONE', #5654, #12142 ) ;
#11613=CARTESIAN_POINT ( 'NONE',  ( -2.500000000000000000, -1.035533905932739307, -1.450000000000000400 ) ) ;
#11628=CARTESIAN_POINT ( 'NONE',  ( 2.500000000000000000, 3.061616997868383141E-16, -0.1999999978150504010 ) ) ;
#11635=EDGE_CURVE ( 'NONE', #3215, #7968, #3188, .T. ) ;
#11637=CARTESIAN_POINT ( 'NONE',  ( 0.8561741729129463963, -2.066987299999999195, 0.7000000010924749549 ) ) ;
#11640=CARTESIAN_POINT ( 'NONE',  ( -2.500000000000000000, 0.000000000000000000, 1.000000002184949777 ) ) ;
#11643=CARTESIAN_POINT ( 'NONE',  ( -2.508389872690818034, 0.2012129740817172052, -2.499130957106830753 ) ) ;
#11653=CARTESIAN_POINT ( 'NONE',  ( 1.767766952966368654, 1.767766952966369098, -1.800000000000000044 ) ) ;
#11660=UNCERTAINTY_MEASURE_WITH_UNIT (LENGTH_MEASURE( 1.000000000000000082E-05 ), #1945, 'distance_accuracy_value', 'NONE');
#11663=CARTESIAN_POINT ( 'NONE',  ( -0.8561741729129455081, 2.066987299999999639, -1.299999998907525267 ) ) ;
#11675=EDGE_CURVE ( 'NONE', #6066, #5999, #408, .T. ) ;
#11677=STYLED_ITEM ( 'NONE', ( #9788 ), #5230 ) ;
#11694=CARTESIAN_POINT ( 'NONE',  ( -2.500000000000000000, 0.000000000000000000, 1.000000002184949777 ) ) ;
#11698=CARTESIAN_POINT ( 'NONE',  ( -0.8561741729129455081, 2.066987299999999639, -2.699999998907525178 ) ) ;
#11705=ORIENTED_EDGE ( 'NONE', *, *, #9722, .F. ) ;
#11707=CARTESIAN_POINT ( 'NONE',  ( 2.500000000000000444, 1.035533905932737975, -0.9499999978150506230 ) ) ;
#11711=CARTESIAN_POINT ( 'NONE',  ( 1.035533905932739085, -2.500000000000000000, -1.243000000021849960 ) ) ;
#11714=CARTESIAN_POINT ( 'NONE',  ( 2.066987300000000083, -0.8561741729129449530, 0.8000000010924747107 ) ) ;
#11719=CARTESIAN_POINT ( 'NONE',  ( -1.370134448080163825, 2.110273492104576043, -2.498966192944565456 ) ) ;
#11729=CARTESIAN_POINT ( 'NONE',  ( 1.767766952966369320, -1.767766952966368654, -2.000000000000000444 ) ) ;
#11732=DIRECTION ( 'NONE',  ( 0.000000000000000000, 0.000000000000000000, -1.000000000000000000 ) ) ;
#11756=FACE_OUTER_BOUND ( 'NONE', #5362, .T. ) ;
#11767=CARTESIAN_POINT ( 'NONE',  ( -1.767766952966368432, -1.767766952966369320, -0.4999999978150501123 ) ) ;
#11771=CARTESIAN_POINT ( 'NONE',  ( -2.066987299999999639, 0.8561741729129452860, -2.599999998907525089 ) ) ;
#11772=AXIS2_PLACEMENT_3D ( 'NONE', #3095, #2125, #4524 ) ;
#11775=ORIENTED_EDGE ( 'NONE', *, *, #11675, .F. ) ;
#11781=CARTESIAN_POINT ( 'NONE',  ( -1.530808498934191571E-16, 2.500000000000000000, 0.8000000021849495990 ) ) ;
#11785=CARTESIAN_POINT ( 'NONE',  ( 4.592425496802573972E-16, -2.500000000000000000, -0.4930000000218495715 ) ) ;
#11789=CARTESIAN_POINT ( 'NONE',  ( -0.8561741729129458411, -2.066987299999999195, 1.400000001092474911 ) ) ;
#11794=VERTEX_POINT ( 'NONE', #4543 ) ;
#11803=CARTESIAN_POINT ( 'NONE',  ( -2.500000000000000000, -1.035533905932739307, -1.349999997815050090 ) ) ;
#11804=CARTESIAN_POINT ( 'NONE',  ( -1.767766952966368432, -1.767766952966369320, 1.000000000000000000 ) ) ;
#11808=EDGE_CURVE ( 'NONE', #3801, #10844, #6328, .T. ) ;
#11823=EDGE_CURVE ( 'NONE', #15063, #3801, #12903, .T. ) ;
#11835=VECTOR ( 'NONE', #7692, 1000.000000000000000 ) ;
#11839=CARTESIAN_POINT ( 'NONE',  ( -1.767766952966369098, 1.767766952966369098, 0.1000000021849497545 ) ) ;
#11843=CARTESIAN_POINT ( 'NONE',  ( 2.066987300000000083, -0.8561741729129449530, -2.199999998907525178 ) ) ;
#11853=CARTESIAN_POINT ( 'NONE',  ( -2.500000000000000000, -1.035533905932739307, -2.149999997815051245 ) ) ;
#11857=CARTESIAN_POINT ( 'NONE',  ( -1.767766952966369098, 1.767766952966369098, -0.7930000000218494494 ) ) ;
#11860=CARTESIAN_POINT ( 'NONE',  ( -0.8561741729129455081, 2.066987299999999639, -0.4999999989075253337 ) ) ;
#11866=ORIENTED_EDGE ( 'NONE', *, *, #201, .F. ) ;
#11881=CARTESIAN_POINT ( 'NONE',  ( -1.767766952966368432, -1.767766952966369320, -2.200000000000000178 ) ) ;
#11891=DIRECTION ( 'NONE',  ( 0.000000000000000000, 0.000000000000000000, -1.000000000000000000 ) ) ;
#11900=CARTESIAN_POINT ( 'NONE',  ( -1.461580736456472795, 1.461580736456472795, -2.849999998907525089 ) ) ;
#11901=CARTESIAN_POINT ( 'NONE',  ( 0.8561741729129463963, -2.066987299999999195, 1.700000001092474733 ) ) ;
#11909=CARTESIAN_POINT ( 'NONE',  ( 2.066987299999999639, 0.8561741729129456191, -0.4999999989075253892 ) ) ;
#11924=CARTESIAN_POINT ( 'NONE',  ( 1.035533905932737531, 2.500000000000000444, -0.8499999978150500901 ) ) ;
#11933=EDGE_CURVE ( 'NONE', #2475, #9302, #7935, .T. ) ;
#11939=CARTESIAN_POINT ( 'NONE',  ( -1.767766952966368432, -1.767766952966369320, -1.299999997815050712 ) ) ;
#11944=CARTESIAN_POINT ( 'NONE',  ( -1.767766952966369098, 1.767766952966369098, 0.8069999999781504174 ) ) ;
#11947=CARTESIAN_POINT ( 'NONE',  ( -2.066987299999999639, 0.8561741729129452860, 2.200000001092475177 ) ) ;
#11951=ORIENTED_EDGE ( 'NONE', *, *, #1242, .F. ) ;
#11953=DIRECTION ( 'NONE',  ( -1.000000000000000000, 0.000000000000000000, 0.000000000000000000 ) ) ;
#11959=EDGE_CURVE ( 'NONE', #2808, #1290, #6377, .T. ) ;
#11967=CARTESIAN_POINT ( 'NONE',  ( -1.084202172485504434E-16, 3.464101615137754830, -2.500000000000000000 ) ) ;
#11973=ORIENTED_EDGE ( 'NONE', *, *, #11067, .T. ) ;
#11983=CARTESIAN_POINT ( 'NONE',  ( 2.066987300000000083, -0.8561741729129449530, -0.5999999989075250895 ) ) ;
#11991=CARTESIAN_POINT ( 'NONE',  ( 2.066987299999999639, 0.8561741729129456191, 1.100000001092475088 ) ) ;
#11992=AXIS2_PLACEMENT_3D ( 'NONE', #3651, #2135, #9635 ) ;
#11993=PLANE ( 'NONE',  #4159 ) ;
#12007=CARTESIAN_POINT ( 'NONE',  ( 2.500000000000000000, 3.061616997868383141E-16, -0.1999999978150501789 ) ) ;
#12009=LINE ( 'NONE', #10904, #1858 ) ;
#12012=DIRECTION ( 'NONE',  ( 0.000000000000000000, 0.000000000000000000, -1.000000000000000000 ) ) ;
#12022=CARTESIAN_POINT ( 'NONE',  ( -0.8561741729129455081, 2.066987299999999639, 1.100000001092475088 ) ) ;
#12027=CARTESIAN_POINT ( 'NONE',  ( 1.035533905932737531, 2.500000000000000444, -1.743000000021849960 ) ) ;
#12030=CARTESIAN_POINT ( 'NONE',  ( -2.066987299999999639, 0.000000000000000000, 2.250000001092474999 ) ) ;
#12033=DIRECTION ( 'NONE',  ( -1.000000000000000000, 0.000000000000000000, 0.000000000000000000 ) ) ;
#12034=ORIENTED_EDGE ( 'NONE', *, *, #7108, .T. ) ;
#12046=DIRECTION ( 'NONE',  ( -1.000000000000000000, 0.000000000000000000, 0.000000000000000000 ) ) ;
#12059=CARTESIAN_POINT ( 'NONE',  ( -2.500000000000000000, 0.000000000000000000, -0.7000000000000000666 ) ) ;
#12062=DIRECTION ( 'NONE',  ( 0.000000000000000000, 0.000000000000000000, -1.000000000000000000 ) ) ;
#12065=CARTESIAN_POINT ( 'NONE',  ( -2.066987299999999639, 0.000000000000000000, -0.1499999989075253282 ) ) ;
#12069=CARTESIAN_POINT ( 'NONE',  ( 2.500000000000000444, -1.035533905932737309, -0.3500000000000000333 ) ) ;
#12073=CARTESIAN_POINT ( 'NONE',  ( -2.066987299999999639, 0.000000000000000000, 1.450000001092474955 ) ) ;
#12088=CARTESIAN_POINT ( 'NONE',  ( -3.000000000000000444, -1.732050807568878081, -2.500000000000000000 ) ) ;
#12098=CARTESIAN_POINT ( 'NONE',  ( -1.530808498934191571E-16, 2.500000000000000000, -2.399999997815050801 ) ) ;
#12102=CARTESIAN_POINT ( 'NONE',  ( 1.767766952966369320, -1.767766952966368654, 0.3999999999999997446 ) ) ;
#12105=CARTESIAN_POINT ( 'NONE',  ( 0.8561741729129463963, -2.066987299999999195, 1.700000001092474733 ) ) ;
#12110=VERTEX_POINT ( 'NONE', #6921 ) ;
#12119=ADVANCED_FACE ( 'NONE', ( #6996 ), #3397, .T. ) ;
#12142=VECTOR ( 'NONE', #4535, 1000.000000000000000 ) ;
#12145=CARTESIAN_POINT ( 'NONE',  ( -2.066987299999999195, -0.8561741729129466183, -0.09999999890752520049 ) ) ;
#12149=FACE_OUTER_BOUND ( 'NONE', #9342, .T. ) ;
#12151=CARTESIAN_POINT ( 'NONE',  ( -0.8561741729129458411, -2.066987299999999195, 1.600000001092474866 ) ) ;
#12152=CARTESIAN_POINT ( 'NONE',  ( 2.999999999999999556, 1.732050807568877859, -2.500000000000000000 ) ) ;
#12159=SURFACE_STYLE_FILL_AREA ( #3724 ) ;
#12167=CARTESIAN_POINT ( 'NONE',  ( 1.767766952966369320, -1.767766952966368654, -2.699999997815051067 ) ) ;
#12170=DIRECTION ( 'NONE',  ( -0.8660254037844400399, 0.000000000000000000, 0.4999999999999975020 ) ) ;
#12180=CARTESIAN_POINT ( 'NONE',  ( -1.530808498934191571E-16, 2.500000000000000000, -1.599999997815050534 ) ) ;
#12184=CARTESIAN_POINT ( 'NONE',  ( -2.500000000000000000, 0.000000000000000000, 2.500000000000000000 ) ) ;
#12187=CARTESIAN_POINT ( 'NONE',  ( 3.796994071234844259E-16, -2.066987299999999639, -1.749999998907525223 ) ) ;
#12214=DIRECTION ( 'NONE',  ( 0.000000000000000000, 0.000000000000000000, 1.000000000000000000 ) ) ;
#12220=CARTESIAN_POINT ( 'NONE',  ( -0.8561741729129455081, 2.066987299999999639, 0.5000000010924747773 ) ) ;
#12241=CARTESIAN_POINT ( 'NONE',  ( 1.035533905932739085, -2.500000000000000000, 0.3500000000000000333 ) ) ;
#12243=CARTESIAN_POINT ( 'NONE',  ( -2.500000000000000000, -1.035533905932739307, -2.949999997815051067 ) ) ;
#12248=DIRECTION ( 'NONE',  ( -1.000000000000000000, 0.000000000000000000, 0.000000000000000000 ) ) ;
#12257=CARTESIAN_POINT ( 'NONE',  ( -1.461580736456472351, -1.461580736456473018, -1.849999998907525534 ) ) ;
#12258=FACE_OUTER_BOUND ( 'NONE', #1915, .T. ) ;
#12261=CARTESIAN_POINT ( 'NONE',  ( -1.530808498934191571E-16, 2.500000000000000000, 2.299999999999999822 ) ) ;
#12265=CARTESIAN_POINT ( 'NONE',  ( -2.066987299999999639, 0.000000000000000000, -1.149999998907525356 ) ) ;
#12295=EDGE_CURVE ( 'NONE', #26, #1214, #8034, .T. ) ;
#12296=CARTESIAN_POINT ( 'NONE',  ( 3.796994071234844259E-16, -2.066987299999999639, -2.349999998907525089 ) ) ;
#12306=CARTESIAN_POINT ( 'NONE',  ( -2.066987299999999639, 0.000000000000000000, 0.4500000010924747329 ) ) ;
#12314=ADVANCED_FACE ( 'NONE', ( #2086 ), #6959, .T. ) ;
#12321=CARTESIAN_POINT ( 'NONE',  ( 0.4831378333609244180, 2.500000000000000000, -3.223327956010960449 ) ) ;
#12334=CARTESIAN_POINT ( 'NONE',  ( -0.8561741729129455081, 2.066987299999999639, -0.4999999989075253337 ) ) ;
#12336=CARTESIAN_POINT ( 'NONE',  ( -1.084202172485504434E-16, 3.464101615137754830, -5.500000000000000000 ) ) ;
#12340=CARTESIAN_POINT ( 'NONE',  ( 2.500000000000000444, -1.035533905932737309, 0.4499999999999998446 ) ) ;
#12344=CARTESIAN_POINT ( 'NONE',  ( 3.796994071234844259E-16, -2.066987299999999639, -0.7499999989075251117 ) ) ;
#12350=EDGE_CURVE ( 'NONE', #26, #3801, #4805, .T. ) ;
#12374=CARTESIAN_POINT ( 'NONE',  ( 2.500000000000000444, 1.035533905932737975, 1.350000000000000089 ) ) ;
#12379=CARTESIAN_POINT ( 'NONE',  ( 1.767766952966369320, -1.767766952966368654, -0.4000000000000001887 ) ) ;
#12382=CARTESIAN_POINT ( 'NONE',  ( 3.796994071234844259E-16, -2.066987299999999639, -2.349999998907525089 ) ) ;
#12386=CARTESIAN_POINT ( 'NONE',  ( -3.827021247335478803E-16, 2.500000000000000000, -2.500000000000000000 ) ) ;
#12404=EDGE_CURVE ( 'NONE', #786, #9805, #14416, .T. ) ;
#12405=ORIENTED_EDGE ( 'NONE', *, *, #4301, .F. ) ;
#12414=VECTOR ( 'NONE', #3781, 1000.000000000000000 ) ;
#12415=CARTESIAN_POINT ( 'NONE',  ( 2.066987300000000083, -0.8561741729129449530, -0.7999999989075252671 ) ) ;
#12419=CARTESIAN_POINT ( 'NONE',  ( -1.767766952966368432, -1.767766952966369320, 0.2000000000000000944 ) ) ;
#12422=CARTESIAN_POINT ( 'NONE',  ( -1.265664690411614835E-16, 2.066987299999999639, -0.3499999989075254225 ) ) ;
#12435=CARTESIAN_POINT ( 'NONE',  ( -1.265664690411614835E-16, 2.066987299999999639, -2.749999998907525001 ) ) ;
#12456=CARTESIAN_POINT ( 'NONE',  ( 1.767766952966369320, -1.767766952966368654, 1.199999999999999956 ) ) ;
#12462=CARTESIAN_POINT ( 'NONE',  ( 0.8561741729129465073, -2.066987299999999195, -2.299999998907525267 ) ) ;
#12463=CARTESIAN_POINT ( 'NONE',  ( 1.035533905932739085, -2.500000000000000000, -2.749999997815050445 ) ) ;
#12464=CARTESIAN_POINT ( 'NONE',  ( 2.066987299999999639, 2.531329380823229670E-16, 0.05000000109247476621 ) ) ;
#12491=CARTESIAN_POINT ( 'NONE',  ( -1.265664690411614835E-16, 2.066987299999999639, -2.149999998907525800 ) ) ;
#12496=CARTESIAN_POINT ( 'NONE',  ( 2.500000000000000444, 1.035533905932737975, -1.850000000000000533 ) ) ;
#12500=CARTESIAN_POINT ( 'NONE',  ( -1.461580736456472351, -1.461580736456473018, -0.04999999890752505893 ) ) ;
#12512=EDGE_CURVE ( 'NONE', #4630, #5531, #9671, .T. ) ;
#12533=CARTESIAN_POINT ( 'NONE',  ( -0.8561741729129458411, -2.066987299999999195, -2.399999998907525356 ) ) ;
#12542=CARTESIAN_POINT ( 'NONE',  ( -2.066987299999999195, -0.8561741729129467293, -1.699999998907525400 ) ) ;
#12545=EDGE_CURVE ( 'NONE', #5531, #5264, #11609, .T. ) ;
#12570=CARTESIAN_POINT ( 'NONE',  ( 2.066987299999999639, 2.531329380823229670E-16, 0.8500000010924746441 ) ) ;
#12573=CARTESIAN_POINT ( 'NONE',  ( -2.500000000000000000, 0.000000000000000000, -1.500000000000000000 ) ) ;
#12579=CARTESIAN_POINT ( 'NONE',  ( -1.265664690411614835E-16, 2.066987299999999639, 1.250000001092474777 ) ) ;
#12592=CARTESIAN_POINT ( 'NONE',  ( -1.767766952966368432, -1.767766952966369320, 1.806999999978150528 ) ) ;
#12600=CARTESIAN_POINT ( 'NONE',  ( -1.785019455104270181, -1.755996401752895286, -2.500026767917371107 ) ) ;
#12611=CARTESIAN_POINT ( 'NONE',  ( -2.500000000000000000, -1.035533905932739307, 1.750000000000000222 ) ) ;
#12617=UNCERTAINTY_MEASURE_WITH_UNIT (LENGTH_MEASURE( 1.000000000000000082E-05 ), #9056, 'distance_accuracy_value', 'NONE');
#12621=CARTESIAN_POINT ( 'NONE',  ( 2.066987299999999639, 0.8561741729129456191, 1.700000001092474733 ) ) ;
#12653=CARTESIAN_POINT ( 'NONE',  ( 2.500000000000000444, 1.035533905932737975, -0.2500000000000002220 ) ) ;
#12657=CARTESIAN_POINT ( 'NONE',  ( -1.530808498934191571E-16, 2.500000000000000000, -2.562499999726881139 ) ) ;
#12659=CARTESIAN_POINT ( 'NONE',  ( -2.066987299999999195, -0.8561741729129466183, -0.8999999989075251339 ) ) ;
#12669=CARTESIAN_POINT ( 'NONE',  ( -2.500000000000000444, 1.035533905932737753, 0.9500000021849496212 ) ) ;
#12674=APPLICATION_CONTEXT ( 'automotive_design' ) ;
#12691=CARTESIAN_POINT ( 'NONE',  ( 1.767766952966368654, 1.767766952966369098, -0.2000000000000000944 ) ) ;
#12699=CARTESIAN_POINT ( 'NONE',  ( -0.8561741729129455081, 2.066987299999999639, -0.4999999989075253892 ) ) ;
#12700=EDGE_CURVE ( 'NONE', #8455, #1570, #7431, .T. ) ;
#12716=ORIENTED_EDGE ( 'NONE', *, *, #7862, .F. ) ;
#12725=VECTOR ( 'NONE', #10309, 1000.000000000000000 ) ;
#12726=CARTESIAN_POINT ( 'NONE',  ( 2.500000000000000000, 3.061616997868383141E-16, 1.400000002184949910 ) ) ;
#12729=CARTESIAN_POINT ( 'NONE',  ( 0.8561741729129451750, 2.066987299999999639, -1.999999998907525223 ) ) ;
#12731=CARTESIAN_POINT ( 'NONE',  ( 0.000000000000000000, 0.000000000000000000, 2.500000000000000000 ) ) ;
#12737=CARTESIAN_POINT ( 'NONE',  ( 0.000000000000000000, 0.000000000000000000, 2.500000000000000000 ) ) ;
#12740=CARTESIAN_POINT ( 'NONE',  ( -2.500000000000000000, -1.035533905932739307, 1.050000002184949599 ) ) ;
#12752=CARTESIAN_POINT ( 'NONE',  ( 0.9998469633096263021, -2.309553665790732957, -2.499997523255642840 ) ) ;
#12760=CARTESIAN_POINT ( 'NONE',  ( 2.500000000000000444, -1.035533905932737309, 0.4499999999999998446 ) ) ;
#12768=AXIS2_PLACEMENT_3D ( 'NONE', #5777, #3220, #2342 ) ;
#12770=CARTESIAN_POINT ( 'NONE',  ( -2.066987299999999639, 0.8561741729129455081, -1.999999998907525001 ) ) ;
#12792=EDGE_CURVE ( 'NONE', #13528, #9302, #13887, .T. ) ;
#12795=EDGE_CURVE ( 'NONE', #1214, #4630, #2029, .T. ) ;
#12802=CARTESIAN_POINT ( 'NONE',  ( 1.035533905932739085, -2.500000000000000000, -1.250000000000000222 ) ) ;
#12803=CARTESIAN_POINT ( 'NONE',  ( -2.500000000000000000, 0.000000000000000000, -1.500000000000000000 ) ) ;
#12808=B_SPLINE_CURVE_WITH_KNOTS ( 'NONE', 1,
 ( #4277, #11203 ),
 .UNSPECIFIED., .F., .F.,
 ( 2, 2 ),
 ( 0.000000000000000000, 1.000000000000000000 ),
 .UNSPECIFIED. ) ;
#12810=ORIENTED_EDGE ( 'NONE', *, *, #3396, .F. ) ;
#12814=ORIENTED_EDGE ( 'NONE', *, *, #12795, .T. ) ;
#12816=CARTESIAN_POINT ( 'NONE',  ( -1.530808498934191571E-16, 2.500000000000000000, 2.184949486963572163E-09 ) ) ;
#12821=CARTESIAN_POINT ( 'NONE',  ( 4.592425496802573972E-16, -2.500000000000000000, 1.906999999978150617 ) ) ;
#12824=CARTESIAN_POINT ( 'NONE',  ( -2.066987299999999195, -0.8561741729129466183, 1.300000001092474600 ) ) ;
#12830=CLOSED_SHELL ( 'NONE', ( #15313, #13856, #6588, #1649, #11389, #9063, #12119, #5629, #14562, #289, #2231, #12314, #5245, #14336, #12929, #3611, #14292, #1320, #2667, #9598, #7008, #4845, #7987, #9833, #10797, #1846, #13407, #3280, #720, #6007 ) ) ;
#12834=LINE ( 'NONE', #13952, #14996 ) ;
#12839=CARTESIAN_POINT ( 'NONE',  ( 1.259047450927248679, 2.184465970885645092, -2.500000000000000444 ) ) ;
#12840=CARTESIAN_POINT ( 'NONE',  ( 1.500000000000000444, 1.836970198721030427E-16, -5.500000000000000000 ) ) ;
#12841=CARTESIAN_POINT ( 'NONE',  ( -1.035533905932737753, 2.500000000000000444, -0.8500000000000001998 ) ) ;
#12850=CARTESIAN_POINT ( 'NONE',  ( 2.066987299999999639, 0.8561741729129456191, -0.6999999989075255113 ) ) ;
#12861=VECTOR ( 'NONE', #9299, 1000.000000000000000 ) ;
#12865=CARTESIAN_POINT ( 'NONE',  ( 1.767766952966369320, -1.767766952966368654, 1.300000002184949821 ) ) ;
#12874=CARTESIAN_POINT ( 'NONE',  ( -1.035533905932737753, 2.500000000000000444, 0.05000000218494983495 ) ) ;
#12878=CARTESIAN_POINT ( 'NONE',  ( 1.035533905932737531, 2.500000000000000444, 0.7500000021849496656 ) ) ;
#12883=CARTESIAN_POINT ( 'NONE',  ( -0.8561741729129458411, -2.066987299999999195, -2.399999998907525356 ) ) ;
#12887=VERTEX_POINT ( 'NONE', #13233 ) ;
#12895=FACE_OUTER_BOUND ( 'NONE', #2903, .T. ) ;
#12902=CARTESIAN_POINT ( 'NONE',  ( 1.035533905932737531, 2.500000000000000444, 0.6569999999781506173 ) ) ;
#12903=( BOUNDED_CURVE ( )  B_SPLINE_CURVE ( 2, ( #6861, #4462, #2064, #2221, #13209, #3578, #2139, #8370, #873 ),
 .UNSPECIFIED., .F., .F. ) 
 B_SPLINE_CURVE_WITH_KNOTS ( ( 3, 2, 2, 2, 3 ),
 ( 0.2142857142857142738, 0.2321428571428571508, 0.2500000000000000000, 0.2678571428571428492, 0.2857142857142856984 ),
 .UNSPECIFIED. ) 
 CURVE ( )  GEOMETRIC_REPRESENTATION_ITEM ( )  RATIONAL_B_SPLINE_CURVE ( ( 1.000000000000000000, 0.9238795325112867385, 1.000000000000000000, 0.9238795325112867385, 1.000000000000000000, 0.9238795325112867385, 1.000000000000000000, 0.9238795325112867385, 1.000000000000000000 ) ) 
 REPRESENTATION_ITEM ( '' )  );
#12905=EDGE_CURVE ( 'NONE', #2808, #13777, #2088, .T. ) ;
#12906=CARTESIAN_POINT ( 'NONE',  ( -0.8561741729129455081, 2.066987299999999639, 1.900000001092474688 ) ) ;
#12910=VECTOR ( 'NONE', #5106, 1000.000000000000000 ) ;
#12912=CARTESIAN_POINT ( 'NONE',  ( -1.472388569876015740, -2.039937050886111880, -2.501127800403732504 ) ) ;
#12922=CARTESIAN_POINT ( 'NONE',  ( 2.500000000000000444, -1.035533905932737309, -1.949999999999999956 ) ) ;
#12924=PRESENTATION_STYLE_ASSIGNMENT (( #5545 ) ) ;
#12925=CARTESIAN_POINT ( 'NONE',  ( -1.767766952966369098, 1.767766952966369098, 1.700000002184949732 ) ) ;
#12929=ADVANCED_FACE ( 'NONE', ( #5842 ), #3602, .T. ) ;
#12931=CARTESIAN_POINT ( 'NONE',  ( 1.461580736456472573, 1.461580736456472795, -0.6499999989075253559 ) ) ;
#12948=CARTESIAN_POINT ( 'NONE',  ( 2.500000000000000000, 3.061616997868383141E-16, 0.6000000021849497545 ) ) ;
#12960=CARTESIAN_POINT ( 'NONE',  ( -1.530808498934191571E-16, 2.500000000000000000, 0.8000000021849498211 ) ) ;
#12963=CARTESIAN_POINT ( 'NONE',  ( -1.530808498934191571E-16, 2.500000000000000000, 0.6999999999999998446 ) ) ;
#12973=CARTESIAN_POINT ( 'NONE',  ( 1.035533905932739085, -2.500000000000000000, 1.250000002184949555 ) ) ;
#12977=CARTESIAN_POINT ( 'NONE',  ( 1.767766952966369320, -1.767766952966368654, -1.993000000021850182 ) ) ;
#12980=CARTESIAN_POINT ( 'NONE',  ( 1.461580736456472573, 1.461580736456472795, 0.1500000010924747995 ) ) ;
#12997=CARTESIAN_POINT ( 'NONE',  ( -1.035533905932738197, -2.500000000000000000, -2.150000000000000355 ) ) ;
#13000=SURFACE_STYLE_FILL_AREA ( #4583 ) ;
#13035=CARTESIAN_POINT ( 'NONE',  ( -2.500000000000000000, 0.000000000000000000, 0.2000000021849497878 ) ) ;
#13039=CARTESIAN_POINT ( 'NONE',  ( -1.767766952966369098, 1.767766952966369098, -1.499999997815050001 ) ) ;
#13043=CARTESIAN_POINT ( 'NONE',  ( -1.461580736456472795, 1.461580736456472795, -2.649999998907524912 ) ) ;
#13052=CARTESIAN_POINT ( 'NONE',  ( -1.461580736456472795, 1.461580736456472795, 1.950000001092474733 ) ) ;
#13056=CARTESIAN_POINT ( 'NONE',  ( 2.500000000000000000, 3.061616997868383141E-16, 0.5069999999781504840 ) ) ;
#13067=ORIENTED_EDGE ( 'NONE', *, *, #12905, .F. ) ;
#13072=CARTESIAN_POINT ( 'NONE',  ( 2.500000000000000000, 3.061616997868383141E-16, 2.500000000000000000 ) ) ;
#13073=CARTESIAN_POINT ( 'NONE',  ( 0.000000000000000000, 0.000000000000000000, 2.500000000000000000 ) ) ;
#13104=CARTESIAN_POINT ( 'NONE',  ( -1.461580736456472795, 1.461580736456472795, 0.5500000010924748217 ) ) ;
#13109=ORIENTED_EDGE ( 'NONE', *, *, #3396, .T. ) ;
#13116=CARTESIAN_POINT ( 'NONE',  ( -1.035533905932737753, 2.500000000000000444, -1.549999997815050268 ) ) ;
#13122=ORIENTED_EDGE ( 'NONE', *, *, #5703, .F. ) ;
#13132=CARTESIAN_POINT ( 'NONE',  ( -2.500000000000000000, -1.035533905932739307, -2.949999997815051067 ) ) ;
#13137=CARTESIAN_POINT ( 'NONE',  ( -1.035533905932737753, 2.500000000000000444, -0.8430000000218496048 ) ) ;
#13139=CARTESIAN_POINT ( 'NONE',  ( 3.796994071234844259E-16, -2.066987299999999639, -0.1499999989075253282 ) ) ;
#13144=ORIENTED_EDGE ( 'NONE', *, *, #1143, .F. ) ;
#13146=AXIS2_PLACEMENT_3D ( 'NONE', #9785, #13433, #3799 ) ;
#13158=CARTESIAN_POINT ( 'NONE',  ( -1.767766952966368432, -1.767766952966369320, -1.299999997815050490 ) ) ;
#13178=CARTESIAN_POINT ( 'NONE',  ( 1.461580736456473018, -1.461580736456472573, 1.750000001092474999 ) ) ;
#13188=CARTESIAN_POINT ( 'NONE',  ( -0.8561741729129455081, 2.066987299999999639, 1.300000001092475044 ) ) ;
#13193=FACE_OUTER_BOUND ( 'NONE', #5105, .T. ) ;
#13206=CARTESIAN_POINT ( 'NONE',  ( -1.530808498934191571E-16, 2.500000000000000000, 2.184949703804006660E-09 ) ) ;
#13209=CARTESIAN_POINT ( 'NONE',  ( 4.592425496802573972E-16, -2.500000000000000000, 1.100000000000000089 ) ) ;
#13215=ORIENTED_EDGE ( 'NONE', *, *, #12792, .T. ) ;
#13218=CARTESIAN_POINT ( 'NONE',  ( -1.035533905932738197, -2.500000000000000000, -2.849999997815050978 ) ) ;
#13223=CARTESIAN_POINT ( 'NONE',  ( 2.500000000000000444, 1.035533905932737975, -0.2430000000218497103 ) ) ;
#13226=CARTESIAN_POINT ( 'NONE',  ( 3.796994071234844259E-16, -2.066987299999999639, 1.650000001092474911 ) ) ;
#13233=CARTESIAN_POINT ( 'NONE',  ( -2.500000000000000000, 0.000000000000000000, 0.09999999999999982514 ) ) ;
#13253=DIRECTION ( 'NONE',  ( 1.000000000000000000, 0.000000000000000000, 0.000000000000000000 ) ) ;
#13260=CARTESIAN_POINT ( 'NONE',  ( 2.066987299999999639, 0.8561741729129456191, 1.100000001092475088 ) ) ;
#13267=CARTESIAN_POINT ( 'NONE',  ( 1.461580736456473018, -1.461580736456472573, -0.6499999989075253559 ) ) ;
#13268=VECTOR ( 'NONE', #3300, 1000.000000000000227 ) ;
#13269=CARTESIAN_POINT ( 'NONE',  ( 2.500000000000000000, 3.061616997868383141E-16, 1.300000000000000044 ) ) ;
#13274=ORIENTED_EDGE ( 'NONE', *, *, #11675, .T. ) ;
#13282=CARTESIAN_POINT ( 'NONE',  ( -1.767766952966369098, 1.767766952966369098, -2.299999997815050712 ) ) ;
#13285=CARTESIAN_POINT ( 'NONE',  ( 1.767766952966368654, 1.767766952966369098, 0.6000000000000000888 ) ) ;
#13296=CARTESIAN_POINT ( 'NONE',  ( -2.500000000000000444, 1.035533905932737753, -2.249999997815050445 ) ) ;
#13301=CARTESIAN_POINT ( 'NONE',  ( -2.500000000000000000, 0.000000000000000000, 0.9000000000000000222 ) ) ;
#13303=CARTESIAN_POINT ( 'NONE',  ( 0.8561741729129463963, -2.066987299999999195, -1.699999998907525400 ) ) ;
#13307=EDGE_LOOP ( 'NONE', ( #3100, #11040, #11540, #10261, #7658, #4134 ) ) ;
#13329=FACE_OUTER_BOUND ( 'NONE', #10017, .T. ) ;
#13336=( BOUNDED_CURVE ( )  B_SPLINE_CURVE ( 2, ( #2878, #1905, #13768, #7963, #10350, #6548, #10122, #9166, #12803 ),
 .UNSPECIFIED., .F., .F. ) 
 B_SPLINE_CURVE_WITH_KNOTS ( ( 3, 2, 2, 2, 3 ),
 ( 0.6428571428571429047, 0.6607142857142856984, 0.6785714285714286031, 0.6964285714285713969, 0.7142857142857143016 ),
 .UNSPECIFIED. ) 
 CURVE ( )  GEOMETRIC_REPRESENTATION_ITEM ( )  RATIONAL_B_SPLINE_CURVE ( ( 1.000000000000000000, 0.9238795325112867385, 1.000000000000000000, 0.9238795325112867385, 1.000000000000000000, 0.9238795325112867385, 1.000000000000000000, 0.9238795325112867385, 1.000000000000000000 ) ) 
 REPRESENTATION_ITEM ( '' )  );
#13338=CARTESIAN_POINT ( 'NONE',  ( -1.265664690411614835E-16, 2.066987299999999639, 2.050000001092474822 ) ) ;
#13344=CARTESIAN_POINT ( 'NONE',  ( 3.796994071234844259E-16, -2.066987299999999639, 1.650000001092474911 ) ) ;
#13358=CARTESIAN_POINT ( 'NONE',  ( -1.035533905932737753, 2.500000000000000444, -2.349999997815050090 ) ) ;
#13369=CARTESIAN_POINT ( 'NONE',  ( 1.767766952966369320, -1.767766952966368654, -2.699999997815051067 ) ) ;
#13373=CARTESIAN_POINT ( 'NONE',  ( -1.767766952966369098, 1.767766952966369098, 2.400000000000000355 ) ) ;
#13377=CARTESIAN_POINT ( 'NONE',  ( -0.8561741729129458411, -2.066987299999999195, 1.600000001092474866 ) ) ;
#13378=CARTESIAN_POINT ( 'NONE',  ( -3.827021247335478803E-16, 2.500000000000000000, -2.500000000000000000 ) ) ;
#13380=AXIS2_PLACEMENT_3D ( 'NONE', #1563, #11116, #3792 ) ;
#13381=CARTESIAN_POINT ( 'NONE',  ( 2.999999999999999556, 1.732050807568877859, -5.500000000000000000 ) ) ;
#13388=FACE_OUTER_BOUND ( 'NONE', #8929, .T. ) ;
#13396=B_SPLINE_CURVE_WITH_KNOTS ( 'NONE', 1,
 ( #14209, #3319 ),
 .UNSPECIFIED., .F., .F.,
 ( 2, 2 ),
 ( 0.000000000000000000, 1.000000000000000000 ),
 .UNSPECIFIED. ) ;
#13407=ADVANCED_FACE ( 'NONE', ( #13193 ), #8437, .T. ) ;
#13408=VERTEX_POINT ( 'NONE', #14631 ) ;
#13417=CARTESIAN_POINT ( 'NONE',  ( -0.8561741729129458411, -2.066987299999999195, 0.8000000010924747107 ) ) ;
#13422=( BOUNDED_CURVE ( )  B_SPLINE_CURVE ( 2, ( #9451, #8021, #10489, #10640, #776, #15343, #15418, #4517, #14368 ),
 .UNSPECIFIED., .F., .F. ) 
 B_SPLINE_CURVE_WITH_KNOTS ( ( 3, 2, 2, 2, 3 ),
 ( 0.3571428571428571508, 0.3750000000000000000, 0.3928571428571428492, 0.4107142857142856984, 0.4285714285714285476 ),
 .UNSPECIFIED. ) 
 CURVE ( )  GEOMETRIC_REPRESENTATION_ITEM ( )  RATIONAL_B_SPLINE_CURVE ( ( 1.000000000000000000, 0.9238795325112867385, 1.000000000000000000, 0.9238795325112867385, 1.000000000000000000, 0.9238795325112867385, 1.000000000000000000, 0.9238795325112867385, 1.000000000000000000 ) ) 
 REPRESENTATION_ITEM ( '' )  );
#13426=CARTESIAN_POINT ( 'NONE',  ( 0.8561741729129452860, 2.066987299999999639, 0.4000000010924748550 ) ) ;
#13433=DIRECTION ( 'NONE',  ( -1.000000000000000000, -6.123233995736782060E-17, 0.000000000000000000 ) ) ;
#13436=DIRECTION ( 'NONE',  ( -1.000000000000000000, 0.000000000000000000, 0.000000000000000000 ) ) ;
#13443=CARTESIAN_POINT ( 'NONE',  ( 2.500000000000000000, 3.061616997868383141E-16, -2.599999997815050534 ) ) ;
#13455=CARTESIAN_POINT ( 'NONE',  ( -1.461580736456472351, -1.461580736456473018, -1.049999998907525489 ) ) ;
#13459=CARTESIAN_POINT ( 'NONE',  ( 1.035533905932739085, -2.500000000000000000, 0.3500000000000000333 ) ) ;
#13463=CARTESIAN_POINT ( 'NONE',  ( 1.461580736456473018, -1.461580736456472573, -0.8499999989075254225 ) ) ;
#13466=VERTEX_POINT ( 'NONE', #2371 ) ;
#13478=DIRECTION ( 'NONE',  ( 0.000000000000000000, 0.000000000000000000, -1.000000000000000000 ) ) ;
#13488=CARTESIAN_POINT ( 'NONE',  ( -1.767766952966369098, 1.767766952966369098, -0.7999999999999999334 ) ) ;
#13492=CARTESIAN_POINT ( 'NONE',  ( 2.066987299999999639, 2.531329380823229670E-16, -0.5499999989075250451 ) ) ;
#13515=DIRECTION ( 'NONE',  ( 0.000000000000000000, -1.000000000000000000, 0.000000000000000000 ) ) ;
#13516=CARTESIAN_POINT ( 'NONE',  ( -1.084202172485504434E-15, -3.464101615137755275, -5.500000000000000000 ) ) ;
#13527=CARTESIAN_POINT ( 'NONE',  ( 2.500000000000000000, 3.061616997868383141E-16, 2.500000000000000000 ) ) ;
#13528=VERTEX_POINT ( 'NONE', #12386 ) ;
#13529=CARTESIAN_POINT ( 'NONE',  ( 0.8561741729129451750, 2.066987299999999639, 0.2000000010924747329 ) ) ;
#13533=CARTESIAN_POINT ( 'NONE',  ( 2.500000000000000444, -1.035533905932737309, 1.250000000000000222 ) ) ;
#13537=CARTESIAN_POINT ( 'NONE',  ( -0.8561741729129455081, 2.066987299999999639, -2.899999998907526244 ) ) ;
#13566=CARTESIAN_POINT ( 'NONE',  ( -2.500000000000000444, 1.035533905932737753, 1.649999999999999911 ) ) ;
#13571=PLANE ( 'NONE',  #5280 ) ;
#13574=CARTESIAN_POINT ( 'NONE',  ( 1.461580736456473018, -1.461580736456472573, -2.249999998907525445 ) ) ;
#13592=CARTESIAN_POINT ( 'NONE',  ( 1.767766984964215471, 1.767766920968521616, -2.500000000000000444 ) ) ;
#13603=CARTESIAN_POINT ( 'NONE',  ( -2.066987299999999195, -0.8561741729129466183, -1.899999998907525800 ) ) ;
#13607=CARTESIAN_POINT ( 'NONE',  ( 1.035533905932739085, -2.500000000000000000, 1.150000000000000133 ) ) ;
#13610=CARTESIAN_POINT ( 'NONE',  ( 1.461580736456473018, -1.461580736456472573, 0.1500000010924746052 ) ) ;
#13641=CARTESIAN_POINT ( 'NONE',  ( 2.500000000000000444, -1.035533905932737309, 1.250000000000000222 ) ) ;
#13649=CARTESIAN_POINT ( 'NONE',  ( -1.461580736456472795, 1.461580736456472795, -2.649999998907524912 ) ) ;
#13654=AXIS2_PLACEMENT_3D ( 'NONE', #8479, #8308, #11953 ) ;
#13664=CARTESIAN_POINT ( 'NONE',  ( 2.500000000000000000, 3.061616997868383141E-16, 0.5000000000000000000 ) ) ;
#13679=CYLINDRICAL_SURFACE ( 'NONE', #11145, 2.500000000000000000 ) ;
#13684=CARTESIAN_POINT ( 'NONE',  ( 0.8561741729129463963, -2.066987299999999195, -1.699999998907525400 ) ) ;
#13686=CARTESIAN_POINT ( 'NONE',  ( -1.035533905932737753, 2.500000000000000444, -1.649999999999999911 ) ) ;
#13689=CARTESIAN_POINT ( 'NONE',  ( 1.767766952966368654, 1.767766952966369098, -1.000000000000000000 ) ) ;
#13693=CARTESIAN_POINT ( 'NONE',  ( -0.8561741729129455081, 2.066987299999999639, 0.5000000010924747773 ) ) ;
#13732=CARTESIAN_POINT ( 'NONE',  ( -1.767766952966369098, 1.767766952966369098, 2.400000000000000355 ) ) ;
#13736=CARTESIAN_POINT ( 'NONE',  ( -1.035533905932738197, -2.500000000000000000, -2.049999997815050268 ) ) ;
#13738=CARTESIAN_POINT ( 'NONE',  ( -2.066987299999999639, 0.8561741729129455081, -1.799999998907525045 ) ) ;
#13739=CARTESIAN_POINT ( 'NONE',  ( 2.500000000000000444, -1.035533905932737309, -2.649999997815050357 ) ) ;
#13763=CARTESIAN_POINT ( 'NONE',  ( 2.066987299999999639, 0.8561741729129456191, 0.1000000010924746996 ) ) ;
#13767=CARTESIAN_POINT ( 'NONE',  ( -2.500000000000000000, -1.035533905932739307, -2.250000000000000444 ) ) ;
#13768=CARTESIAN_POINT ( 'NONE',  ( 1.767766952966369320, -1.767766952966368654, -1.200000000000000178 ) ) ;
#13772=CARTESIAN_POINT ( 'NONE',  ( 0.8561741729129463963, -2.066987299999999195, -0.6999999989075250673 ) ) ;
#13777=VERTEX_POINT ( 'NONE', #8252 ) ;
#13778=ORIENTED_EDGE ( 'NONE', *, *, #8137, .T. ) ;
#13779=CARTESIAN_POINT ( 'NONE',  ( -2.500000000000000000, 0.000000000000000000, 1.000000002184949777 ) ) ;
#13788=CARTESIAN_POINT ( 'NONE',  ( 1.767766952966369320, -1.767766952966368654, 1.206999999978150440 ) ) ;
#13795=CARTESIAN_POINT ( 'NONE',  ( 1.767766952966369320, -1.767766952966368654, 0.5000000021849496656 ) ) ;
#13804=CARTESIAN_POINT ( 'NONE',  ( 4.592425496802573972E-16, -2.500000000000000000, 1.899999999999999911 ) ) ;
#13810=CARTESIAN_POINT ( 'NONE',  ( -2.500000000000000000, 0.000000000000000000, 2.500000000000000000 ) ) ;
#13813=CARTESIAN_POINT ( 'NONE',  ( 2.066987299999999639, 0.8561741729129456191, 0.9000000010924746885 ) ) ;
#13821=VECTOR ( 'NONE', #4758, 1000.000000000000000 ) ;
#13841=CARTESIAN_POINT ( 'NONE',  ( 2.500000000000000000, 3.061616997868383141E-16, -1.900000000000000133 ) ) ;
#13843=CARTESIAN_POINT ( 'NONE',  ( -2.500000000000000000, -0.4783542904563624076, 1.823096990497731884 ) ) ;
#13845=CARTESIAN_POINT ( 'NONE',  ( -2.500000000000000000, 0.000000000000000000, -0.5999999978150503122 ) ) ;
#13846=CARTESIAN_POINT ( 'NONE',  ( -1.461580736456472351, -1.461580736456473018, -1.649999998907525356 ) ) ;
#13856=ADVANCED_FACE ( 'NONE', ( #13329 ), #7220, .T. ) ;
#13857=CARTESIAN_POINT ( 'NONE',  ( -2.500000000000000000, 0.000000000000000000, 1.000000002184949777 ) ) ;
#13878=CARTESIAN_POINT ( 'NONE',  ( 2.500000000000000000, 3.061616997868383141E-16, 2.100000000000000089 ) ) ;
#13879=CARTESIAN_POINT ( 'NONE',  ( -1.265664690411614835E-16, 2.066987299999999639, -1.949999998907525622 ) ) ;
#13887=B_SPLINE_CURVE_WITH_KNOTS ( 'NONE', 3,
 ( #3852, #8726, #5456, #15155, #11719, #10226, #1857, #10303, #6807, #15310, #822, #11643, #10380, #9267, #6731, #745, #510, #5687, #12600, #12912, #3058, #15077, #4250, #11563, #9120, #8964, #7909, #12752, #10534, #7834, #11409, #5380, #659, #1699, #5532, #15230, #4333, #7754, #1933, #3137, #9190, #13949 ),
 .UNSPECIFIED., .F., .F.,
 ( 4, 2, 2, 2, 2, 2, 2, 2, 2, 2, 2, 2, 2, 2, 2, 2, 2, 2, 2, 2, 4 ),
 ( 0.000000000000000000, 0.06250000000000002776, 0.1250000000000000555, 0.1562500000000000555, 0.1875000000000000833, 0.2500000000000001110, 0.3125000000000001110, 0.3750000000000001665, 0.4062500000000001665, 0.4375000000000001110, 0.5000000000000001110, 0.5625000000000000000, 0.5937500000000000000, 0.6250000000000000000, 0.6875000000000001110, 0.7500000000000001110, 0.8125000000000001110, 0.8437500000000001110, 0.8750000000000001110, 0.9375000000000001110, 1.000000000000000000 ),
 .UNSPECIFIED. ) ;
#13889=CARTESIAN_POINT ( 'NONE',  ( -1.265664690411614835E-16, 2.066987299999999639, -1.349999998907525534 ) ) ;
#13912=AXIS2_PLACEMENT_3D ( 'NONE', #3412, #7089, #10741 ) ;
#13915=CARTESIAN_POINT ( 'NONE',  ( -2.066987299999999195, -0.8561741729129466183, -2.699999998907525178 ) ) ;
#13920=CARTESIAN_POINT ( 'NONE',  ( -1.767766952966369098, 1.767766952966369098, -2.399999999999999911 ) ) ;
#13924=CARTESIAN_POINT ( 'NONE',  ( 0.8561741729129451750, 2.066987299999999639, 1.200000001092474733 ) ) ;
#13935=CARTESIAN_POINT ( 'NONE',  ( 1.035533905932739085, -2.500000000000000000, -1.149999997815050357 ) ) ;
#13948=ORIENTED_EDGE ( 'NONE', *, *, #1709, .F. ) ;
#13949=CARTESIAN_POINT ( 'NONE',  ( 1.767766984964215471, 1.767766920968521616, -2.500000000000000444 ) ) ;
#13952=CARTESIAN_POINT ( 'NONE',  ( -2.500000000000000000, 0.000000000000000000, 2.500000000000000000 ) ) ;
#13961=CARTESIAN_POINT ( 'NONE',  ( 1.767766952966369320, -1.767766952966368654, -1.200000000000000178 ) ) ;
#13963=CARTESIAN_POINT ( 'NONE',  ( -1.530808498934191571E-16, 2.500000000000000000, 1.600000002184949865 ) ) ;
#13972=CARTESIAN_POINT ( 'NONE',  ( 0.8561741729129465073, -2.066987299999999195, -0.09999999890752520049 ) ) ;
#14000=CARTESIAN_POINT ( 'NONE',  ( -1.530808498934191571E-16, 2.500000000000000000, -2.500000000000000000 ) ) ;
#14012=DIRECTION ( 'NONE',  ( 0.000000000000000000, 0.000000000000000000, 1.000000000000000000 ) ) ;
#14017=CARTESIAN_POINT ( 'NONE',  ( 1.767766952966368654, 1.767766952966369098, 1.500000002184949777 ) ) ;
#14021=CARTESIAN_POINT ( 'NONE',  ( 1.767766952966369320, -1.767766952966368654, 2.006999999978150484 ) ) ;
#14039=CARTESIAN_POINT ( 'NONE',  ( -2.500000000000000444, 1.035533905932737753, -1.549999999999999600 ) ) ;
#14041=CARTESIAN_POINT ( 'NONE',  ( 1.767766952966368654, 1.767766952966369098, 1.500000002184949777 ) ) ;
#14046=CARTESIAN_POINT ( 'NONE',  ( 1.461580736456473018, -1.461580736456472573, -0.8499999989075254225 ) ) ;
#14051=DIRECTION ( 'NONE',  ( 0.000000000000000000, 0.000000000000000000, 1.000000000000000000 ) ) ;
#14074=CARTESIAN_POINT ( 'NONE',  ( 4.592425496802573972E-16, -2.500000000000000000, 0.4000000021849499099 ) ) ;
#14088=CARTESIAN_POINT ( 'NONE',  ( 1.767766952966368654, 1.767766952966369098, 0.7000000021849496212 ) ) ;
#14089=VECTOR ( 'NONE', #6142, 1000.000000000000000 ) ;
#14094=CARTESIAN_POINT ( 'NONE',  ( -2.500000000000000000, 0.000000000000000000, 2.506999999978150484 ) ) ;
#14097=CARTESIAN_POINT ( 'NONE',  ( -2.066987299999999639, 0.000000000000000000, 2.050000001092474822 ) ) ;
#14103=CARTESIAN_POINT ( 'NONE',  ( -2.500000000000000000, -1.035533905932739307, 0.2500000021849497212 ) ) ;
#14113=CARTESIAN_POINT ( 'NONE',  ( -1.767766952966368432, -1.767766952966369320, 1.800000000000000044 ) ) ;
#14115=CARTESIAN_POINT ( 'NONE',  ( 2.500000000000000444, -1.035533905932737309, -1.150000000000000133 ) ) ;
#14122=CARTESIAN_POINT ( 'NONE',  ( -0.8561741729129455081, 2.066987299999999639, -2.899999998907526244 ) ) ;
#14127=ORIENTED_EDGE ( 'NONE', *, *, #14600, .F. ) ;
#14138=DIRECTION ( 'NONE',  ( -1.000000000000000000, 0.000000000000000000, 0.000000000000000000 ) ) ;
#14153=CARTESIAN_POINT ( 'NONE',  ( 2.500000000000000444, -1.035533905932737309, 0.5500000021849498211 ) ) ;
#14168=CARTESIAN_POINT ( 'NONE',  ( -1.035533905932737753, 2.500000000000000444, 0.8500000021849496434 ) ) ;
#14169=VECTOR ( 'NONE', #13515, 1000.000000000000000 ) ;
#14173=CARTESIAN_POINT ( 'NONE',  ( 2.500000000000000444, -1.035533905932737309, -1.943000000021849472 ) ) ;
#14175=CARTESIAN_POINT ( 'NONE',  ( -1.461580736456472351, -1.461580736456473018, -0.2499999989075251672 ) ) ;
#14178=CARTESIAN_POINT ( 'NONE',  ( -1.035533905932737753, 2.500000000000000444, 0.8500000021849498655 ) ) ;
#14183=EDGE_LOOP ( 'NONE', ( #7260, #3315, #14899, #14276 ) ) ;
#14193=CARTESIAN_POINT ( 'NONE',  ( 4.592425496802573972E-16, -2.500000000000000000, -2.100000000000000089 ) ) ;
#14200=CARTESIAN_POINT ( 'NONE',  ( 1.461580736456472573, 1.461580736456472795, -2.249999998907525001 ) ) ;
#14201=AXIS2_PLACEMENT_3D ( 'NONE', #6680, #11513, #1651 ) ;
#14209=CARTESIAN_POINT ( 'NONE',  ( -1.265664690411614835E-16, 2.066987299999999639, -2.949999998907525178 ) ) ;
#14228=CARTESIAN_POINT ( 'NONE',  ( 1.035533905932739085, -2.500000000000000000, 1.250000002184949999 ) ) ;
#14231=CARTESIAN_POINT ( 'NONE',  ( 1.035533905932737531, 2.500000000000000444, 0.6500000000000000222 ) ) ;
#14235=ORIENTED_EDGE ( 'NONE', *, *, #10572, .T. ) ;
#14239=ORIENTED_EDGE ( 'NONE', *, *, #1976, .F. ) ;
#14240=CARTESIAN_POINT ( 'NONE',  ( 2.500000000000000000, 3.061616997868383141E-16, -1.799999997815050712 ) ) ;
#14243=DIRECTION ( 'NONE',  ( 0.000000000000000000, 0.000000000000000000, -1.000000000000000000 ) ) ;
#14245=CARTESIAN_POINT ( 'NONE',  ( 1.035533905932739085, -2.500000000000000000, 0.3569999999781505173 ) ) ;
#14249=CARTESIAN_POINT ( 'NONE',  ( -2.066987299999999639, 0.8561741729129452860, -0.3999999989075250784 ) ) ;
#14252=CARTESIAN_POINT ( 'NONE',  ( -1.767766952966369098, 1.767766952966369098, 0.9000000021849497989 ) ) ;
#14276=ORIENTED_EDGE ( 'NONE', *, *, #8137, .F. ) ;
#14287=CYLINDRICAL_SURFACE ( 'NONE', #930, 2.500000000000000000 ) ;
#14291=CARTESIAN_POINT ( 'NONE',  ( 0.8561741729129465073, -2.066987299999999195, -0.6999999989075250673 ) ) ;
#14292=ADVANCED_FACE ( 'NONE', ( #1917, #5595 ), #726, .T. ) ;
#14302=CARTESIAN_POINT ( 'NONE',  ( 2.500000000000000444, 1.035533905932737975, 0.6500000021849499099 ) ) ;
#14303=CYLINDRICAL_SURFACE ( 'NONE', #13912, 1.500000000000000000 ) ;
#14309=ORIENTED_EDGE ( 'NONE', *, *, #7371, .T. ) ;
#14312=EDGE_LOOP ( 'NONE', ( #14127, #14363, #9189, #8196 ) ) ;
#14315=( BOUNDED_SURFACE ( )  B_SPLINE_SURFACE ( 1, 2, ( 
 ( #9370, #10638, #11589, #3554, #13338, #2595, #9530, #7147, #1318, #3631, #13178, #11901, #2440, #8507, #5872, #8661, #9846, #1009, #14619, #9613, #7227, #4756, #1089, #13260, #11031, #9695, #2277, #4918, #129, #13417, #10719, #8340, #6194, #15577, #4995, #12220, #3708, #8585, #6032, #15654, #2523, #1163, #9774, #14696, #4837, #14451, #2359, #12145, #12065, #7303, #14365, #4677, #3784, #6116, #14532, #3471, #13492, #11983, #52, #8423, #10795, #1244, #10953, #5951, #10878, #10901, #7378, #15013, #366, #213, #519, #5390, #15088, #10237, #4105, #4183, #4020, #3862, #9054, #5314, #6269, #1475, #8896, #286, #13879, #11187, #11419, #7764, #3937, #7528, #6584, #7451, #12296, #12533, #1394, #6509, #8975, #7608, #11108, #5149, #14928 ),
 ( #10159, #11342, #13732, #5232, #2839, #5072, #8813, #9923, #14776, #10078, #1633, #2757, #13804, #2913, #7685, #12611, #8734, #13566, #2676, #10004, #6353, #439, #1707, #12374, #14851, #13641, #12456, #1556, #6433, #11265, #11804, #908, #10622, #5776, #10543, #15485, #15322, #15165, #4581, #833, #1788, #12760, #4422, #11573, #9432, #6740, #6971, #3299, #15241, #3068, #2101, #2992, #7846, #8082, #12691, #2022, #15401, #3146, #6663, #669, #10467, #11495, #4342, #598, #5469, #10312, #4262, #12841, #9199, #3219, #8161, #9130, #9277, #14115, #13961, #7919, #5699, #5543, #1866, #10393, #4497, #14039, #6896, #7999, #1943, #6818, #11653, #755, #5621, #12922, #11729, #9351, #14193, #12997, #11881, #9512, #3691, #6014, #15559, #4980, #4821 ) ),
 .UNSPECIFIED., .F., .F., .F. ) 
 B_SPLINE_SURFACE_WITH_KNOTS ( ( 2, 2 ),
 ( 3, 2, 2, 2, 2, 2, 2, 2, 2, 2, 2, 2, 2, 2, 2, 2, 2, 2, 2, 2, 2, 2, 2, 2, 2, 2, 2, 2, 2, 2, 2, 2, 2, 2, 2, 2, 2, 2, 2, 2, 2, 2, 2, 2, 2, 2, 2, 2, 2, 2, 3 ),
 ( 0.000000000000000000, 1.000000000000000000 ),
 ( 0.000000000000000000, 0.01785714285714285615, 0.03571428571428571230, 0.05357142857142856845, 0.07142857142857142461, 0.08928571428571428770, 0.1071428571428571369, 0.1250000000000000000, 0.1428571428571428492, 0.1607142857142857262, 0.1785714285714285754, 0.1964285714285714246, 0.2142857142857142738, 0.2321428571428571508, 0.2500000000000000000, 0.2678571428571428492, 0.2857142857142856984, 0.3035714285714285476, 0.3214285714285714524, 0.3392857142857143016, 0.3571428571428571508, 0.3750000000000000000, 0.3928571428571428492, 0.4107142857142856984, 0.4285714285714285476, 0.4464285714285714524, 0.4642857142857143016, 0.4821428571428571508, 0.5000000000000000000, 0.5178571428571429047, 0.5357142857142856984, 0.5535714285714286031, 0.5714285714285713969, 0.5892857142857143016, 0.6071428571428570953, 0.6250000000000000000, 0.6428571428571429047, 0.6607142857142856984, 0.6785714285714286031, 0.6964285714285713969, 0.7142857142857143016, 0.7321428571428570953, 0.7500000000000000000, 0.7678571428571429047, 0.7857142857142856984, 0.8035714285714286031, 0.8214285714285713969, 0.8392857142857143016, 0.8571428571428570953, 0.8750000000000000000, 0.8928571428571429047 ),
 .UNSPECIFIED. ) 
 GEOMETRIC_REPRESENTATION_ITEM ( )  RATIONAL_B_SPLINE_SURFACE ( (
 ( 1.000000000000000000, 0.9238795325112867385, 1.000000000000000000, 0.9238795325112867385, 1.000000000000000000, 0.9238795325112867385, 1.000000000000000000, 0.9238795325112867385, 1.000000000000000000, 0.9238795325112867385, 1.000000000000000000, 0.9238795325112867385, 1.000000000000000000, 0.9238795325112867385, 1.000000000000000000, 0.9238795325112867385, 1.000000000000000000, 0.9238795325112867385, 1.000000000000000000, 0.9238795325112867385, 1.000000000000000000, 0.9238795325112867385, 1.000000000000000000, 0.9238795325112867385, 1.000000000000000000, 0.9238795325112867385, 1.000000000000000000, 0.9238795325112867385, 1.000000000000000000, 0.9238795325112867385, 1.000000000000000000, 0.9238795325112867385, 1.000000000000000000, 0.9238795325112867385, 1.000000000000000000, 0.9238795325112867385, 1.000000000000000000, 0.9238795325112867385, 1.000000000000000000, 0.9238795325112867385, 1.000000000000000000, 0.9238795325112867385, 1.000000000000000000, 0.9238795325112867385, 1.000000000000000000, 0.9238795325112867385, 1.000000000000000000, 0.9238795325112867385, 1.000000000000000000, 0.9238795325112867385, 1.000000000000000000, 0.9238795325112867385, 1.000000000000000000, 0.9238795325112867385, 1.000000000000000000, 0.9238795325112867385, 1.000000000000000000, 0.9238795325112867385, 1.000000000000000000, 0.9238795325112867385, 1.000000000000000000, 0.9238795325112867385, 1.000000000000000000, 0.9238795325112867385, 1.000000000000000000, 0.9238795325112867385, 1.000000000000000000, 0.9238795325112867385, 1.000000000000000000, 0.9238795325112867385, 1.000000000000000000, 0.9238795325112867385, 1.000000000000000000, 0.9238795325112867385, 1.000000000000000000, 0.9238795325112867385, 1.000000000000000000, 0.9238795325112867385, 1.000000000000000000, 0.9238795325112867385, 1.000000000000000000, 0.9238795325112867385, 1.000000000000000000, 0.9238795325112867385, 1.000000000000000000, 0.9238795325112867385, 1.000000000000000000, 0.9238795325112867385, 1.000000000000000000, 0.9238795325112867385, 1.000000000000000000, 0.9238795325112867385, 1.000000000000000000, 0.9238795325112867385, 1.000000000000000000, 0.9238795325112867385, 1.000000000000000000, 0.9238795325112867385, 1.000000000000000000, 0.9238795325112867385, 1.000000000000000000),
 ( 1.000000000000000000, 0.9238795325112867385, 1.000000000000000000, 0.9238795325112867385, 1.000000000000000000, 0.9238795325112867385, 1.000000000000000000, 0.9238795325112867385, 1.000000000000000000, 0.9238795325112867385, 1.000000000000000000, 0.9238795325112867385, 1.000000000000000000, 0.9238795325112867385, 1.000000000000000000, 0.9238795325112867385, 1.000000000000000000, 0.9238795325112867385, 1.000000000000000000, 0.9238795325112867385, 1.000000000000000000, 0.9238795325112867385, 1.000000000000000000, 0.9238795325112867385, 1.000000000000000000, 0.9238795325112867385, 1.000000000000000000, 0.9238795325112867385, 1.000000000000000000, 0.9238795325112867385, 1.000000000000000000, 0.9238795325112867385, 1.000000000000000000, 0.9238795325112867385, 1.000000000000000000, 0.9238795325112867385, 1.000000000000000000, 0.9238795325112867385, 1.000000000000000000, 0.9238795325112867385, 1.000000000000000000, 0.9238795325112867385, 1.000000000000000000, 0.9238795325112867385, 1.000000000000000000, 0.9238795325112867385, 1.000000000000000000, 0.9238795325112867385, 1.000000000000000000, 0.9238795325112867385, 1.000000000000000000, 0.9238795325112867385, 1.000000000000000000, 0.9238795325112867385, 1.000000000000000000, 0.9238795325112867385, 1.000000000000000000, 0.9238795325112867385, 1.000000000000000000, 0.9238795325112867385, 1.000000000000000000, 0.9238795325112867385, 1.000000000000000000, 0.9238795325112867385, 1.000000000000000000, 0.9238795325112867385, 1.000000000000000000, 0.9238795325112867385, 1.000000000000000000, 0.9238795325112867385, 1.000000000000000000, 0.9238795325112867385, 1.000000000000000000, 0.9238795325112867385, 1.000000000000000000, 0.9238795325112867385, 1.000000000000000000, 0.9238795325112867385, 1.000000000000000000, 0.9238795325112867385, 1.000000000000000000, 0.9238795325112867385, 1.000000000000000000, 0.9238795325112867385, 1.000000000000000000, 0.9238795325112867385, 1.000000000000000000, 0.9238795325112867385, 1.000000000000000000, 0.9238795325112867385, 1.000000000000000000, 0.9238795325112867385, 1.000000000000000000, 0.9238795325112867385, 1.000000000000000000, 0.9238795325112867385, 1.000000000000000000, 0.9238795325112867385, 1.000000000000000000, 0.9238795325112867385, 1.000000000000000000) ) ) 
 REPRESENTATION_ITEM ( '' )  SURFACE ( )  );
#14317=CARTESIAN_POINT ( 'NONE',  ( -1.035533905932738197, -2.500000000000000000, -1.249999997815050445 ) ) ;
#14321=CARTESIAN_POINT ( 'NONE',  ( -1.035533905932737753, 2.500000000000000444, 0.7569999999781505950 ) ) ;
#14326=CARTESIAN_POINT ( 'NONE',  ( -0.8561741729129458411, -2.066987299999999195, -0.1999999989075254836 ) ) ;
#14327=CARTESIAN_POINT ( 'NONE',  ( -2.500000000000000444, 1.035533905932737753, -2.350000000000000533 ) ) ;
#14336=ADVANCED_FACE ( 'NONE', ( #6557, #15215 ), #805, .T. ) ;
#14363=ORIENTED_EDGE ( 'NONE', *, *, #1853, .T. ) ;
#14365=CARTESIAN_POINT ( 'NONE',  ( -1.461580736456472795, 1.461580736456472795, -0.2499999989075251672 ) ) ;
#14368=CARTESIAN_POINT ( 'NONE',  ( -2.500000000000000000, 0.000000000000000000, -0.5999999978150503122 ) ) ;
#14374=CARTESIAN_POINT ( 'NONE',  ( 1.461580736456472573, 1.461580736456472795, 1.150000001092474911 ) ) ;
#14376=ORIENTED_EDGE ( 'NONE', *, *, #11933, .F. ) ;
#14391=CARTESIAN_POINT ( 'NONE',  ( -2.500000000000000000, -1.035533905932739307, 0.2500000021849496656 ) ) ;
#14399=ORIENTED_EDGE ( 'NONE', *, *, #1804, .F. ) ;
#14404=CARTESIAN_POINT ( 'NONE',  ( -1.035533905932737753, 2.500000000000000444, -3.149999997815050801 ) ) ;
#14410=CARTESIAN_POINT ( 'NONE',  ( -2.500000000000000000, 0.000000000000000000, 0.9069999999781503952 ) ) ;
#14413=CARTESIAN_POINT ( 'NONE',  ( -2.066987299999999195, -0.8561741729129466183, -1.899999998907525800 ) ) ;
#14414=CARTESIAN_POINT ( 'NONE',  ( 2.999999999999999556, -1.732050807568877859, -5.500000000000000000 ) ) ;
#14416=LINE ( 'NONE', #13381, #9270 ) ;
#14418=ORIENTED_EDGE ( 'NONE', *, *, #553, .F. ) ;
#14426=PLANE ( 'NONE',  #8392 ) ;
#14434=FACE_OUTER_BOUND ( 'NONE', #412, .T. ) ;
#14441=EDGE_LOOP ( 'NONE', ( #15413, #5103, #4137, #13144 ) ) ;
#14451=CARTESIAN_POINT ( 'NONE',  ( -0.8561741729129458411, -2.066987299999999195, 1.092474635061568626E-09 ) ) ;
#14461=CARTESIAN_POINT ( 'NONE',  ( 3.796994071234844259E-16, -2.066987299999999639, 0.8500000010924748661 ) ) ;
#14463=DIRECTION ( 'NONE',  ( 0.5000000000000000000, -0.8660254037844387076, 0.000000000000000000 ) ) ;
#14491=CARTESIAN_POINT ( 'NONE',  ( -0.8561741729129458411, -2.066987299999999195, 1.400000001092474911 ) ) ;
#14495=CARTESIAN_POINT ( 'NONE',  ( 1.767766952966368654, 1.767766952966369098, -1.793000000021849338 ) ) ;
#14498=CARTESIAN_POINT ( 'NONE',  ( 1.461580736456473018, -1.461580736456472573, -1.649999998907525356 ) ) ;
#14502=CARTESIAN_POINT ( 'NONE',  ( -2.500000000000000000, 0.000000000000000000, 2.500000000000000000 ) ) ;
#14505=CARTESIAN_POINT ( 'NONE',  ( -1.084202172485504434E-15, -3.464101615137755275, -5.500000000000000000 ) ) ;
#14510=CARTESIAN_POINT ( 'NONE',  ( 2.500000000000000000, 3.061616997868383141E-16, 1.400000002184949910 ) ) ;
#14511=CARTESIAN_POINT ( 'NONE',  ( -2.066987299999999639, 0.000000000000000000, 2.250000001092474999 ) ) ;
#14530=ORIENTED_EDGE ( 'NONE', *, *, #12350, .F. ) ;
#14532=CARTESIAN_POINT ( 'NONE',  ( 1.461580736456472573, 1.461580736456472795, -0.4499999989075252338 ) ) ;
#14536=( BOUNDED_CURVE ( )  B_SPLINE_CURVE ( 2, ( #10140, #14992, #503, #5446, #14833, #6643, #5370, #8954, #6719 ),
 .UNSPECIFIED., .F., .F. ) 
 B_SPLINE_CURVE_WITH_KNOTS ( ( 3, 2, 2, 2, 3 ),
 ( 0.7857142857142856984, 0.8035714285714286031, 0.8214285714285713969, 0.8392857142857143016, 0.8571428571428570953 ),
 .UNSPECIFIED. ) 
 CURVE ( )  GEOMETRIC_REPRESENTATION_ITEM ( )  RATIONAL_B_SPLINE_CURVE ( ( 1.000000000000000000, 0.9238795325112867385, 1.000000000000000000, 0.9238795325112867385, 1.000000000000000000, 0.9238795325112867385, 1.000000000000000000, 0.9238795325112867385, 1.000000000000000000 ) ) 
 REPRESENTATION_ITEM ( '' )  );
#14540=CARTESIAN_POINT ( 'NONE',  ( -2.066987299999999639, 0.8561741729129455081, -0.9999999989075253337 ) ) ;
#14556=CARTESIAN_POINT ( 'NONE',  ( 1.035533905932737531, 2.500000000000000444, -2.449999997815050179 ) ) ;
#14557=CARTESIAN_POINT ( 'NONE',  ( 2.999999999999999556, 1.732050807568877859, -5.500000000000000000 ) ) ;
#14562=ADVANCED_FACE ( 'NONE', ( #3821 ), #13679, .T. ) ;
#14563=ORIENTED_EDGE ( 'NONE', *, *, #11067, .F. ) ;
#14567=ORIENTED_EDGE ( 'NONE', *, *, #10914, .F. ) ;
#14570=CARTESIAN_POINT ( 'NONE',  ( 2.066987299999999639, 0.8561741729129456191, 0.9000000010924746885 ) ) ;
#14572=CARTESIAN_POINT ( 'NONE',  ( -2.500000000000000000, 0.000000000000000000, 0.09999999999999982514 ) ) ;
#14575=CARTESIAN_POINT ( 'NONE',  ( 1.035533905932739085, -2.500000000000000000, -2.043000000021849782 ) ) ;
#14578=CARTESIAN_POINT ( 'NONE',  ( -0.8561741729129455081, 2.066987299999999639, -2.099999998907525089 ) ) ;
#14583=DIRECTION ( 'NONE',  ( 0.000000000000000000, 0.000000000000000000, -1.000000000000000000 ) ) ;
#14600=EDGE_CURVE ( 'NONE', #3437, #12110, #14734, .T. ) ;
#14619=CARTESIAN_POINT ( 'NONE',  ( -1.461580736456472795, 1.461580736456472795, 1.350000001092474644 ) ) ;
#14626=CARTESIAN_POINT ( 'NONE',  ( -1.461580736456472351, -1.461580736456473018, 1.550000001092474822 ) ) ;
#14631=CARTESIAN_POINT ( 'NONE',  ( -3.000000000000000444, -1.732050807568878081, -2.500000000000000000 ) ) ;
#14636=CYLINDRICAL_SURFACE ( 'NONE', #8402, 2.500000000000000000 ) ;
#14643=DIRECTION ( 'NONE',  ( 1.000000000000000000, 0.000000000000000000, 0.000000000000000000 ) ) ;
#14656=CARTESIAN_POINT ( 'NONE',  ( 1.461580736456473018, -1.461580736456472573, 0.7500000010924746663 ) ) ;
#14658=CARTESIAN_POINT ( 'NONE',  ( 1.767766952966368654, 1.767766952966369098, -0.2000000000000000944 ) ) ;
#14660=CARTESIAN_POINT ( 'NONE',  ( -2.500000000000000000, -1.035533905932739307, 0.9499999999999999556 ) ) ;
#14664=CARTESIAN_POINT ( 'NONE',  ( -0.8561741729129455081, 2.066987299999999639, 1.300000001092474822 ) ) ;
#14678=CARTESIAN_POINT ( 'NONE',  ( 2.500000000000000000, 3.061616997868383141E-16, 2.500000000000000000 ) ) ;
#14680=CARTESIAN_POINT ( 'NONE',  ( 1.035533905932737531, 2.500000000000000444, 2.250000000000000888 ) ) ;
#14696=CARTESIAN_POINT ( 'NONE',  ( 0.8561741729129463963, -2.066987299999999195, 0.1000000010924748939 ) ) ;
#14703=CARTESIAN_POINT ( 'NONE',  ( -1.461580736456472351, -1.461580736456473018, -2.449999998907525178 ) ) ;
#14708=CARTESIAN_POINT ( 'NONE',  ( -1.265664690411614835E-16, 2.066987299999999639, 1.050000001092474822 ) ) ;
#14732=AXIS2_PLACEMENT_3D ( 'NONE', #9072, #14950, #4041 ) ;
#14734=LINE ( 'NONE', #13527, #12910 ) ;
#14736=CARTESIAN_POINT ( 'NONE',  ( -2.066987299999999639, 0.8561741729129452860, -0.3999999989075250784 ) ) ;
#14740=CARTESIAN_POINT ( 'NONE',  ( -1.767766952966369098, 1.767766952966369098, 1.599999999999999867 ) ) ;
#14745=CARTESIAN_POINT ( 'NONE',  ( 1.461580736456472573, 1.461580736456472795, -2.249999998907525001 ) ) ;
#14776=CARTESIAN_POINT ( 'NONE',  ( 2.500000000000000000, 3.061616997868383141E-16, 2.100000000000000089 ) ) ;
#14780=FACE_OUTER_BOUND ( 'NONE', #14441, .T. ) ;
#14782=CARTESIAN_POINT ( 'NONE',  ( 2.066987300000000083, -0.8561741729129450640, -2.199999998907525178 ) ) ;
#14784=CARTESIAN_POINT ( 'NONE',  ( 2.066987300000000083, -0.8561741729129450640, 1.600000001092474644 ) ) ;
#14785=VECTOR ( 'NONE', #9427, 1000.000000000000000 ) ;
#14798=CARTESIAN_POINT ( 'NONE',  ( 0.9662756667218489470, 2.500000000000000000, -3.246655914206870275 ) ) ;
#14812=CARTESIAN_POINT ( 'NONE',  ( 0.8561741729129463963, -2.066987299999999195, 0.7000000010924749549 ) ) ;
#14816=CARTESIAN_POINT ( 'NONE',  ( -1.767766952966368432, -1.767766952966369320, 1.800000000000000044 ) ) ;
#14820=CARTESIAN_POINT ( 'NONE',  ( -0.8561741729129458411, -2.066987299999999195, -0.7999999989075252671 ) ) ;
#14832=CARTESIAN_POINT ( 'NONE',  ( -3.000000000000000000, 1.732050807568877415, -2.500000000000000000 ) ) ;
#14833=CARTESIAN_POINT ( 'NONE',  ( 4.592425496802573972E-16, -2.500000000000000000, -2.100000000000000089 ) ) ;
#14851=CARTESIAN_POINT ( 'NONE',  ( 2.500000000000000000, 3.061616997868383141E-16, 1.300000000000000044 ) ) ;
#14858=CARTESIAN_POINT ( 'NONE',  ( -1.265664690411614835E-16, 2.066987299999999639, -1.149999998907525356 ) ) ;
#14865=ORIENTED_EDGE ( 'NONE', *, *, #6920, .F. ) ;
#14888=CARTESIAN_POINT ( 'NONE',  ( -1.461580736456472795, 1.461580736456472795, -2.049999998907525711 ) ) ;
#14893=CARTESIAN_POINT ( 'NONE',  ( 2.500000000000000000, 3.061616997868383141E-16, 1.300000000000000044 ) ) ;
#14896=CARTESIAN_POINT ( 'NONE',  ( 1.461580736456473018, -1.461580736456472573, -0.6499999989075253559 ) ) ;
#14899=ORIENTED_EDGE ( 'NONE', *, *, #9799, .F. ) ;
#14905=EDGE_LOOP ( 'NONE', ( #7795, #9662, #11973, #10030 ) ) ;
#14922=VECTOR ( 'NONE', #8089, 1000.000000000000000 ) ;
#14928=CARTESIAN_POINT ( 'NONE',  ( -1.265664690411614835E-16, 2.066987299999999639, -2.749999998907525001 ) ) ;
#14937=PLANE ( 'NONE',  #13380 ) ;
#14938=CARTESIAN_POINT ( 'NONE',  ( -1.530808498934191571E-16, 2.500000000000000000, -3.199999997815050623 ) ) ;
#14948=EDGE_CURVE ( 'NONE', #13466, #8455, #48, .T. ) ;
#14950=DIRECTION ( 'NONE',  ( 0.000000000000000000, 0.000000000000000000, 1.000000000000000000 ) ) ;
#14951=CARTESIAN_POINT ( 'NONE',  ( 4.592425496802573972E-16, -2.500000000000000000, 0.2999999999999999334 ) ) ;
#14969=CARTESIAN_POINT ( 'NONE',  ( -2.066987299999999639, 0.000000000000000000, -1.949999998907525178 ) ) ;
#14973=CARTESIAN_POINT ( 'NONE',  ( 2.500000000000000444, 1.035533905932737975, 1.450000002184950176 ) ) ;
#14978=CARTESIAN_POINT ( 'NONE',  ( 0.8561741729129463963, -2.066987299999999195, 0.9000000010924746885 ) ) ;
#14992=CARTESIAN_POINT ( 'NONE',  ( 2.500000000000000444, -1.035533905932737309, -1.949999999999999956 ) ) ;
#14996=VECTOR ( 'NONE', #2092, 1000.000000000000000 ) ;
#15013=CARTESIAN_POINT ( 'NONE',  ( -0.8561741729129455081, 2.066987299999999639, -1.099999998907525089 ) ) ;
#15021=CARTESIAN_POINT ( 'NONE',  ( 0.8561741729129465073, -2.066987299999999195, 1.500000001092474555 ) ) ;
#15038=EDGE_CURVE ( 'NONE', #4950, #13528, #10791, .T. ) ;
#15048=CARTESIAN_POINT ( 'NONE',  ( -2.500000000000000444, 1.035533905932737753, -2.350000000000000533 ) ) ;
#15052=CARTESIAN_POINT ( 'NONE',  ( -1.035533905932737753, 2.500000000000000444, -0.7499999978150503344 ) ) ;
#15053=CARTESIAN_POINT ( 'NONE',  ( 2.066987300000000083, -0.8561741729129449530, -1.399999998907525134 ) ) ;
#15057=ORIENTED_EDGE ( 'NONE', *, *, #3458, .T. ) ;
#15063=VERTEX_POINT ( 'NONE', #8658 ) ;
#15070=CARTESIAN_POINT ( 'NONE',  ( 1.767766952966368654, 1.767766952966369098, 2.206999999978150662 ) ) ;
#15077=CARTESIAN_POINT ( 'NONE',  ( -0.6887091348229088528, -2.420707839511175408, -2.499422994081509586 ) ) ;
#15088=CARTESIAN_POINT ( 'NONE',  ( 2.066987299999999639, 2.531329380823229670E-16, -1.349999998907525534 ) ) ;
#15096=CARTESIAN_POINT ( 'NONE',  ( -2.500000000000000000, 0.000000000000000000, -2.999999997815050889 ) ) ;
#15116=ORIENTED_EDGE ( 'NONE', *, *, #11106, .T. ) ;
#15119=ORIENTED_EDGE ( 'NONE', *, *, #6021, .F. ) ;
#15125=CARTESIAN_POINT ( 'NONE',  ( -1.767766952966368432, -1.767766952966369320, -1.400000000000000133 ) ) ;
#15132=CARTESIAN_POINT ( 'NONE',  ( -2.066987299999999195, -0.8561741729129466183, 0.7000000010924749549 ) ) ;
#15138=DIRECTION ( 'NONE',  ( 1.000000000000000000, 0.000000000000000000, 0.000000000000000000 ) ) ;
#15140=ORIENTED_EDGE ( 'NONE', *, *, #11106, .F. ) ;
#15142=CARTESIAN_POINT ( 'NONE',  ( 2.500000000000000444, -1.035533905932737309, -1.049999997815050490 ) ) ;
#15155=CARTESIAN_POINT ( 'NONE',  ( -1.113756821657925000, 2.256897984573015048, -2.499694356362072156 ) ) ;
#15165=CARTESIAN_POINT ( 'NONE',  ( 1.035533905932737531, 2.500000000000000444, 0.6500000000000000222 ) ) ;
#15166=CARTESIAN_POINT ( 'NONE',  ( -1.265664690411614835E-16, 2.066987299999999639, -2.749999998907525001 ) ) ;
#15172=CARTESIAN_POINT ( 'NONE',  ( 0.8561741729129465073, -2.066987299999999195, -1.699999998907525400 ) ) ;
#15204=CARTESIAN_POINT ( 'NONE',  ( -2.500000000000000000, -1.035533905932739307, -0.6500000000000000222 ) ) ;
#15205=CARTESIAN_POINT ( 'NONE',  ( -1.767766952966369098, 1.767766952966369098, 2.400000000000000355 ) ) ;
#15207=CARTESIAN_POINT ( 'NONE',  ( -1.767766952966369098, 1.767766952966369098, -0.6999999978150501789 ) ) ;
#15208=CARTESIAN_POINT ( 'NONE',  ( 1.461580736456472573, 1.461580736456472795, -2.049999998907525267 ) ) ;
#15215=FACE_BOUND ( 'NONE', #44, .T. ) ;
#15216=ORIENTED_EDGE ( 'NONE', *, *, #7543, .F. ) ;
#15217=CARTESIAN_POINT ( 'NONE',  ( -2.500000000000000444, 1.035533905932737753, 1.750000002184949777 ) ) ;
#15221=CARTESIAN_POINT ( 'NONE',  ( 2.500000000000000444, -1.035533905932737309, 2.056999999978150306 ) ) ;
#15224=CARTESIAN_POINT ( 'NONE',  ( 3.796994071234844259E-16, -2.066987299999999639, 1.450000001092474733 ) ) ;
#15228=ORIENTED_EDGE ( 'NONE', *, *, #1713, .F. ) ;
#15230=CARTESIAN_POINT ( 'NONE',  ( 2.503681785030714479, -0.03945699161127848992, -2.499748181185309281 ) ) ;
#15231=ORIENTED_EDGE ( 'NONE', *, *, #355, .T. ) ;
#15235=DIRECTION ( 'NONE',  ( 0.8660254037844385966, -0.4999999999999998890, 0.000000000000000000 ) ) ;
#15241=CARTESIAN_POINT ( 'NONE',  ( -2.500000000000000000, 0.000000000000000000, 0.09999999999999982514 ) ) ;
#15246=STYLED_ITEM ( 'NONE', ( #12924 ), #10501 ) ;
#15251=CARTESIAN_POINT ( 'NONE',  ( -1.265664690411614835E-16, 2.066987299999999639, -2.149999998907525800 ) ) ;
#15255=ORIENTED_EDGE ( 'NONE', *, *, #9844, .F. ) ;
#15267=CARTESIAN_POINT ( 'NONE',  ( 2.500000000000000444, -1.035533905932737309, 1.350000002184949865 ) ) ;
#15269=PRODUCT_DEFINITION_SHAPE ( 'NONE', 'NONE',  #3310 ) ;
#15278=CARTESIAN_POINT ( 'NONE',  ( 1.035533905932737531, 2.500000000000000444, -0.04999999781505021224 ) ) ;
#15282=CARTESIAN_POINT ( 'NONE',  ( 2.500000000000000444, -1.035533905932737309, -0.2499999978150503066 ) ) ;
#15288=ORIENTED_EDGE ( 'NONE', *, *, #1274, .F. ) ;
#15290=ORIENTED_EDGE ( 'NONE', *, *, #11808, .F. ) ;
#15292=VECTOR ( 'NONE', #11493, 1000.000000000000000 ) ;
#15298=CARTESIAN_POINT ( 'NONE',  ( -2.500000000000000000, 0.000000000000000000, -0.5999999978150505342 ) ) ;
#15302=CARTESIAN_POINT ( 'NONE',  ( -1.530808498934191571E-16, 2.500000000000000000, 1.506999999978150706 ) ) ;
#15304=CARTESIAN_POINT ( 'NONE',  ( -0.8561741729129458411, -2.066987299999999195, 0.6000000010924746441 ) ) ;
#15310=CARTESIAN_POINT ( 'NONE',  ( -2.290915817347055849, 1.041596279477050135, -2.500307733819811862 ) ) ;
#15313=ADVANCED_FACE ( 'NONE', ( #7994 ), #5463, .F. ) ;
#15314=CARTESIAN_POINT ( 'NONE',  ( 2.999999999999999556, -1.732050807568877859, -5.500000000000000000 ) ) ;
#15316=DIRECTION ( 'NONE',  ( 0.000000000000000000, 0.000000000000000000, -1.000000000000000000 ) ) ;
#15322=CARTESIAN_POINT ( 'NONE',  ( -1.530808498934191571E-16, 2.500000000000000000, 0.6999999999999998446 ) ) ;
#15332=CARTESIAN_POINT ( 'NONE',  ( -2.066987299999999639, 0.000000000000000000, -2.749999998907525445 ) ) ;
#15343=CARTESIAN_POINT ( 'NONE',  ( -1.035533905932738197, -2.500000000000000000, -0.4499999978150504010 ) ) ;
#15349=CARTESIAN_POINT ( 'NONE',  ( -2.500000000000000000, 0.000000000000000000, 1.000000002184949777 ) ) ;
#15362=CARTESIAN_POINT ( 'NONE',  ( -2.500000000000000444, 1.035533905932737753, -1.449999997815050401 ) ) ;
#15372=VERTEX_POINT ( 'NONE', #14510 ) ;
#15376=CARTESIAN_POINT ( 'NONE',  ( 1.035533905932737531, 2.500000000000000444, -0.04999999781505042734 ) ) ;
#15380=CARTESIAN_POINT ( 'NONE',  ( -1.767766952966368432, -1.767766952966369320, 0.2069999999781506062 ) ) ;
#15383=CARTESIAN_POINT ( 'NONE',  ( -2.066987299999999639, 0.000000000000000000, 0.4500000010924747329 ) ) ;
#15384=EDGE_CURVE ( 'NONE', #1214, #10844, #11009, .T. ) ;
#15396=DIRECTION ( 'NONE',  ( -1.000000000000000000, 0.000000000000000000, 0.000000000000000000 ) ) ;
#15401=CARTESIAN_POINT ( 'NONE',  ( 2.500000000000000000, 3.061616997868383141E-16, -0.2999999999999999334 ) ) ;
#15402=LINE ( 'NONE', #4741, #13268 ) ;
#15403=CARTESIAN_POINT ( 'NONE',  ( 2.500000000000000000, 3.061616997868383141E-16, 1.400000002184949910 ) ) ;
#15408=CARTESIAN_POINT ( 'NONE',  ( -1.461580736456472351, -1.461580736456473018, -0.2499999989075251672 ) ) ;
#15412=CARTESIAN_POINT ( 'NONE',  ( 1.500000000000000000, 1.836970198721029934E-16, 2.500000000000000000 ) ) ;
#15413=ORIENTED_EDGE ( 'NONE', *, *, #8942, .F. ) ;
#15418=CARTESIAN_POINT ( 'NONE',  ( -1.767766952966368432, -1.767766952966369320, -0.4999999978150501123 ) ) ;
#15435=CARTESIAN_POINT ( 'NONE',  ( 2.500000000000000000, 3.061616997868383141E-16, -0.1999999978150501789 ) ) ;
#15440=CARTESIAN_POINT ( 'NONE',  ( 2.500000000000000444, 1.035533905932737975, -0.9499999978150502900 ) ) ;
#15442=CARTESIAN_POINT ( 'NONE',  ( -2.500000000000000000, 0.000000000000000000, 2.500000000000000000 ) ) ;
#15445=CARTESIAN_POINT ( 'NONE',  ( 3.796994071234844259E-16, -2.066987299999999639, -2.349999998907525089 ) ) ;
#15455=CARTESIAN_POINT ( 'NONE',  ( -1.035533905932737753, 2.500000000000000444, 1.650000002184949910 ) ) ;
#15460=CARTESIAN_POINT ( 'NONE',  ( -2.500000000000000444, 1.035533905932737753, -0.7430000000218497380 ) ) ;
#15462=CARTESIAN_POINT ( 'NONE',  ( 2.066987299999999639, 0.8561741729129456191, 0.9000000010924746885 ) ) ;
#15472=ORIENTED_EDGE ( 'NONE', *, *, #12905, .T. ) ;
#15485=CARTESIAN_POINT ( 'NONE',  ( -1.035533905932737753, 2.500000000000000444, 0.7500000000000001110 ) ) ;
#15487=SURFACE_SIDE_STYLE ('',( #13000 ) ) ;
#15497=CARTESIAN_POINT ( 'NONE',  ( 1.767766952966368654, 1.767766952966369098, -1.699999997815050179 ) ) ;
#15504=LINE ( 'NONE', #4683, #14922 ) ;
#15507=CARTESIAN_POINT ( 'NONE',  ( -2.066987299999999639, 0.8561741729129455081, 0.6000000010924748661 ) ) ;
#15508=PLANE ( 'NONE',  #11772 ) ;
#15519=CARTESIAN_POINT ( 'NONE',  ( -1.035533905932737753, 2.500000000000000444, -0.7499999978150503344 ) ) ;
#15523=DIRECTION ( 'NONE',  ( 0.000000000000000000, 0.000000000000000000, -1.000000000000000000 ) ) ;
#15535=CARTESIAN_POINT ( 'NONE',  ( 0.8561741729129451750, 2.066987299999999639, 1.000000001092474555 ) ) ;
#15539=CARTESIAN_POINT ( 'NONE',  ( 1.767766952966369320, -1.767766952966368654, -1.193000000021849472 ) ) ;
#15543=CARTESIAN_POINT ( 'NONE',  ( 0.8561741729129451750, 2.066987299999999639, -0.5999999989075250895 ) ) ;
#15559=CARTESIAN_POINT ( 'NONE',  ( -1.767766952966369098, 1.767766952966369098, -2.399999999999999911 ) ) ;
#15566=( BOUNDED_CURVE ( )  B_SPLINE_CURVE ( 2, ( #2765, #6277, #373, #13739, #4112, #12463, #3869, #6592, #1565, #7773, #15096, #10087, #6441, #1482, #14938 ),
 .UNSPECIFIED., .F., .F. ) 
 B_SPLINE_CURVE_WITH_KNOTS ( ( 3, 2, 2, 2, 2, 2, 2, 3 ),
 ( 0.7678571432794594198, 0.7857142857142856984, 0.8035714285714286031, 0.8214285714285713969, 0.8392857142857143016, 0.8571428571428570953, 0.8750000000000000000, 0.8928571428571429047 ),
 .UNSPECIFIED. ) 
 CURVE ( )  GEOMETRIC_REPRESENTATION_ITEM ( )  RATIONAL_B_SPLINE_CURVE ( ( 1.000000000000000000, 0.9238795325112867385, 1.000000000000000000, 0.9238795325112867385, 1.000000000000000000, 0.9238795325112867385, 1.000000000000000000, 0.9238795325112867385, 1.000000000000000000, 0.9238795325112867385, 1.000000000000000000, 0.9238795325112867385, 1.000000000000000000, 0.9238795325112867385, 1.000000000000000000 ) ) 
 REPRESENTATION_ITEM ( '' )  );
#15572=CARTESIAN_POINT ( 'NONE',  ( 1.767766952966368654, 1.767766952966369098, -1.000000000000000000 ) ) ;
#15576=CARTESIAN_POINT ( 'NONE',  ( -1.461580736456472351, -1.461580736456473018, -2.649999998907525356 ) ) ;
#15577=CARTESIAN_POINT ( 'NONE',  ( -2.066987299999999639, 0.8561741729129452860, 0.6000000010924748661 ) ) ;
#15584=CARTESIAN_POINT ( 'NONE',  ( 2.066987300000000083, -0.8561741729129450640, 1.800000001092475044 ) ) ;
#15600=CARTESIAN_POINT ( 'NONE',  ( 2.500000000000000000, 3.061616997868383141E-16, -1.799999997815050490 ) ) ;
#15607=ORIENTED_EDGE ( 'NONE', *, *, #4301, .T. ) ;
#15612=CARTESIAN_POINT ( 'NONE',  ( -1.767766952966368432, -1.767766952966369320, -2.099999997815050534 ) ) ;
#15616=CARTESIAN_POINT ( 'NONE',  ( 1.767766952966368654, 1.767766952966369098, 0.6069999999781504618 ) ) ;
#15618=CARTESIAN_POINT ( 'NONE',  ( -0.8561741729129458411, -2.066987299999999195, -2.599999998907525534 ) ) ;
#15622=VERTEX_POINT ( 'NONE', #5212 ) ;
#15654=CARTESIAN_POINT ( 'NONE',  ( 2.066987299999999639, 0.8561741729129456191, 0.3000000010924747662 ) ) ;
#15663=CARTESIAN_POINT ( 'NONE',  ( -1.461580736456472351, -1.461580736456473018, -0.04999999890752505893 ) ) ;
#15685=EDGE_LOOP ( 'NONE', ( #6262, #2727, #685, #8654 ) ) ;
#15691=CARTESIAN_POINT ( 'NONE',  ( 1.767766952966368654, 1.767766952966369098, -1.699999997815050401 ) ) ;
#15696=CARTESIAN_POINT ( 'NONE',  ( -2.500000000000000000, -1.035533905932739307, 0.1569999999781505062 ) ) ;
#15700=CARTESIAN_POINT ( 'NONE',  ( -1.265664690411614835E-16, 2.066987299999999639, -1.349999998907525534 ) ) ;
#15711=CIRCLE ( 'NONE', #10123, 2.500000000000000000 ) ;
ENDSEC;
END-ISO-10303-21;
